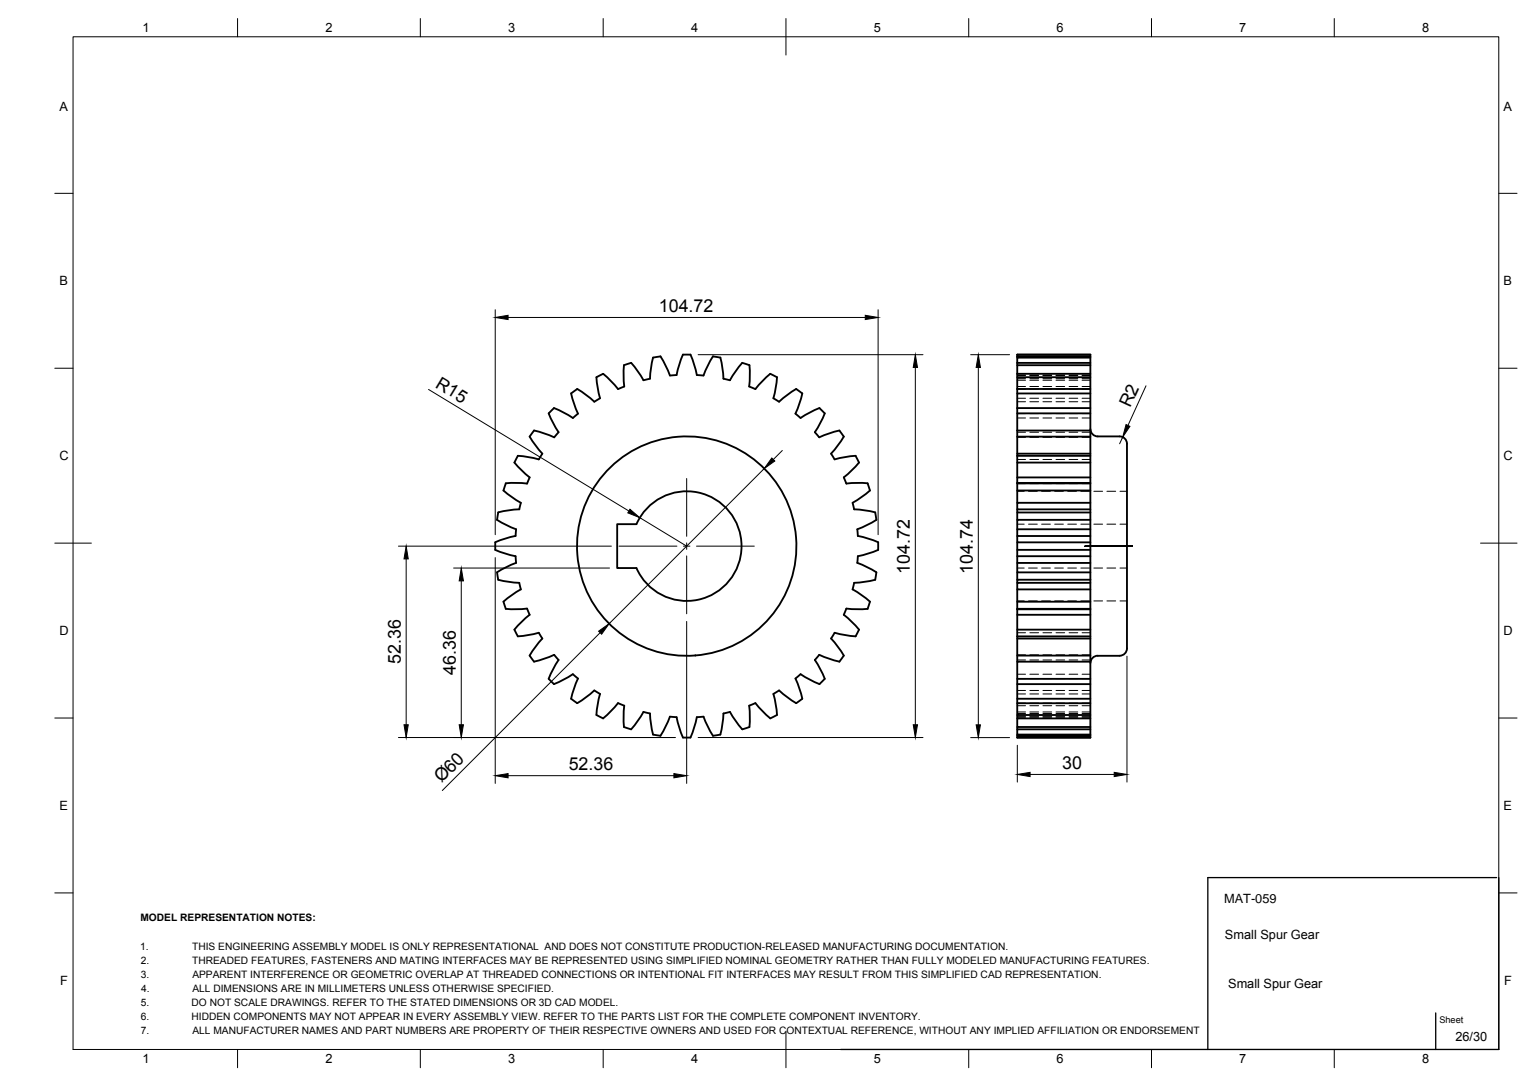
ISO-10303-21;
HEADER;
/* Generated by software containing ST-Developer
 * from STEP Tools, Inc. (www.steptools.com) 
 */

FILE_DESCRIPTION(
/* description */ ('', 'CAx-IF Rec.Pracs.---Representation and Presentation of Product Manufa
cturing Information (PMI)---4.0---2014-10-13'),
/* implementation_level */ '2;1');

FILE_NAME(
/* name */ 'Small Spur Gear.step',
/* time_stamp */ '2026-10-28T23:00:48+01:00',
/* author */ (''),
/* organization */ (''),
/* preprocessor_version */ 'ST-DEVELOPER v20.2',
/* originating_system */ 'Autodesk Translation Framework v15.17.0.0',
/* authorisation */ '');

FILE_SCHEMA (('AP242_MANAGED_MODEL_BASED_3D_ENGINEERING_MIM_LF { 1 0 10303 442 2 1 4 }'));
ENDSEC;

DATA;
#10=MECHANICAL_DESIGN_GEOMETRIC_PRESENTATION_REPRESENTATION('',(#997),#61811);
#908=TOROIDAL_SURFACE('',#36745,28.,2.);
#909=TOROIDAL_SURFACE('',#36754,32.,2.);
#933=SHAPE_REPRESENTATION_RELATIONSHIP('SRR','None',#61994,#958);
#958=ADVANCED_BREP_SHAPE_REPRESENTATION('',(#1036),#61807);
#997=STYLED_ITEM('',(#62149),#1036);
#1036=MANIFOLD_SOLID_BREP('Body1',#33827);
#1589=CYLINDRICAL_SURFACE('',#36750,30.);
#1590=CYLINDRICAL_SURFACE('',#36920,15.);
#1591=CYLINDRICAL_SURFACE('',#36923,46.875);
#1592=CYLINDRICAL_SURFACE('',#36925,27.0484525317045);
#1593=CYLINDRICAL_SURFACE('',#36927,27.0484525317045);
#1594=CYLINDRICAL_SURFACE('',#36929,46.875);
#1595=CYLINDRICAL_SURFACE('',#36931,27.0484525317045);
#1596=CYLINDRICAL_SURFACE('',#36933,27.0484525317045);
#1597=CYLINDRICAL_SURFACE('',#36935,46.875);
#1598=CYLINDRICAL_SURFACE('',#36937,27.0484525317045);
#1599=CYLINDRICAL_SURFACE('',#36939,27.0484525317045);
#1600=CYLINDRICAL_SURFACE('',#36941,46.875);
#1601=CYLINDRICAL_SURFACE('',#36943,27.0484525317045);
#1602=CYLINDRICAL_SURFACE('',#36945,27.0484525317045);
#1603=CYLINDRICAL_SURFACE('',#36947,46.875);
#1604=CYLINDRICAL_SURFACE('',#36949,27.0484525317045);
#1605=CYLINDRICAL_SURFACE('',#36951,27.0484525317045);
#1606=CYLINDRICAL_SURFACE('',#36953,46.875);
#1607=CYLINDRICAL_SURFACE('',#36955,27.0484525317045);
#1608=CYLINDRICAL_SURFACE('',#36957,27.0484525317045);
#1609=CYLINDRICAL_SURFACE('',#36959,46.875);
#1610=CYLINDRICAL_SURFACE('',#36961,27.0484525317045);
#1611=CYLINDRICAL_SURFACE('',#36963,27.0484525317045);
#1612=CYLINDRICAL_SURFACE('',#36965,46.875);
#1613=CYLINDRICAL_SURFACE('',#36967,27.0484525317045);
#1614=CYLINDRICAL_SURFACE('',#36969,27.0484525317045);
#1615=CYLINDRICAL_SURFACE('',#36971,46.875);
#1616=CYLINDRICAL_SURFACE('',#36973,27.0484525317045);
#1617=CYLINDRICAL_SURFACE('',#36975,27.0484525317045);
#1618=CYLINDRICAL_SURFACE('',#36977,46.875);
#1619=CYLINDRICAL_SURFACE('',#36979,27.0484525317045);
#1620=CYLINDRICAL_SURFACE('',#36981,27.0484525317045);
#1621=CYLINDRICAL_SURFACE('',#36983,46.875);
#1622=CYLINDRICAL_SURFACE('',#36985,27.0484525317045);
#1623=CYLINDRICAL_SURFACE('',#36987,27.0484525317045);
#1624=CYLINDRICAL_SURFACE('',#36989,46.875);
#1625=CYLINDRICAL_SURFACE('',#36991,27.0484525317045);
#1626=CYLINDRICAL_SURFACE('',#36993,27.0484525317045);
#1627=CYLINDRICAL_SURFACE('',#36995,46.875);
#1628=CYLINDRICAL_SURFACE('',#36997,27.0484525317045);
#1629=CYLINDRICAL_SURFACE('',#36999,27.0484525317045);
#1630=CYLINDRICAL_SURFACE('',#37001,46.875);
#1631=CYLINDRICAL_SURFACE('',#37003,27.0484525317045);
#1632=CYLINDRICAL_SURFACE('',#37005,27.0484525317045);
#1633=CYLINDRICAL_SURFACE('',#37007,46.875);
#1634=CYLINDRICAL_SURFACE('',#37009,27.0484525317045);
#1635=CYLINDRICAL_SURFACE('',#37011,27.0484525317045);
#1636=CYLINDRICAL_SURFACE('',#37013,46.875);
#1637=CYLINDRICAL_SURFACE('',#37015,27.0484525317045);
#1638=CYLINDRICAL_SURFACE('',#37017,27.0484525317045);
#1639=CYLINDRICAL_SURFACE('',#37019,46.875);
#1640=CYLINDRICAL_SURFACE('',#37021,27.0484525317045);
#1641=CYLINDRICAL_SURFACE('',#37023,27.0484525317045);
#1642=CYLINDRICAL_SURFACE('',#37025,46.875);
#1643=CYLINDRICAL_SURFACE('',#37027,27.0484525317045);
#1644=CYLINDRICAL_SURFACE('',#37029,27.0484525317045);
#1645=CYLINDRICAL_SURFACE('',#37031,46.875);
#1646=CYLINDRICAL_SURFACE('',#37033,27.0484525317045);
#1647=CYLINDRICAL_SURFACE('',#37035,27.0484525317045);
#1648=CYLINDRICAL_SURFACE('',#37037,46.875);
#1649=CYLINDRICAL_SURFACE('',#37039,27.0484525317045);
#1650=CYLINDRICAL_SURFACE('',#37041,27.0484525317045);
#1651=CYLINDRICAL_SURFACE('',#37043,46.875);
#1652=CYLINDRICAL_SURFACE('',#37045,27.0484525317045);
#1653=CYLINDRICAL_SURFACE('',#37047,27.0484525317045);
#1654=CYLINDRICAL_SURFACE('',#37049,46.875);
#1655=CYLINDRICAL_SURFACE('',#37051,27.0484525317045);
#1656=CYLINDRICAL_SURFACE('',#37053,27.0484525317045);
#1657=CYLINDRICAL_SURFACE('',#37055,46.875);
#1658=CYLINDRICAL_SURFACE('',#37057,27.0484525317045);
#1659=CYLINDRICAL_SURFACE('',#37059,27.0484525317045);
#1660=CYLINDRICAL_SURFACE('',#37061,46.875);
#1661=CYLINDRICAL_SURFACE('',#37063,27.0484525317045);
#1662=CYLINDRICAL_SURFACE('',#37065,27.0484525317045);
#1663=CYLINDRICAL_SURFACE('',#37067,46.875);
#1664=CYLINDRICAL_SURFACE('',#37069,27.0484525317045);
#1665=CYLINDRICAL_SURFACE('',#37071,27.0484525317045);
#1666=CYLINDRICAL_SURFACE('',#37073,46.875);
#1667=CYLINDRICAL_SURFACE('',#37075,27.0484525317045);
#1668=CYLINDRICAL_SURFACE('',#37077,27.0484525317045);
#1669=CYLINDRICAL_SURFACE('',#37079,46.875);
#1670=CYLINDRICAL_SURFACE('',#37081,27.0484525317045);
#1671=CYLINDRICAL_SURFACE('',#37083,27.0484525317045);
#1672=CYLINDRICAL_SURFACE('',#37085,46.875);
#1673=CYLINDRICAL_SURFACE('',#37087,27.0484525317045);
#1674=CYLINDRICAL_SURFACE('',#37089,27.0484525317045);
#1675=CYLINDRICAL_SURFACE('',#37091,46.875);
#1676=CYLINDRICAL_SURFACE('',#37093,27.0484525317045);
#1677=CYLINDRICAL_SURFACE('',#37095,27.0484525317045);
#1678=CYLINDRICAL_SURFACE('',#37097,46.875);
#1679=CYLINDRICAL_SURFACE('',#37099,27.0484525317045);
#1680=CYLINDRICAL_SURFACE('',#37101,27.0484525317045);
#1681=CYLINDRICAL_SURFACE('',#37103,46.875);
#1682=CYLINDRICAL_SURFACE('',#37105,27.0484525317045);
#1683=CYLINDRICAL_SURFACE('',#37107,27.0484525317045);
#1684=CYLINDRICAL_SURFACE('',#37109,46.875);
#1685=CYLINDRICAL_SURFACE('',#37111,27.0484525317045);
#1686=CYLINDRICAL_SURFACE('',#37113,27.0484525317045);
#1687=CYLINDRICAL_SURFACE('',#37115,46.875);
#1688=CYLINDRICAL_SURFACE('',#37117,27.0484525317045);
#1689=CYLINDRICAL_SURFACE('',#37119,27.0484525317045);
#1690=CYLINDRICAL_SURFACE('',#37121,46.875);
#1691=CYLINDRICAL_SURFACE('',#37123,27.0484525317045);
#1692=CYLINDRICAL_SURFACE('',#37125,27.0484525317045);
#1693=CYLINDRICAL_SURFACE('',#37127,46.875);
#1694=CYLINDRICAL_SURFACE('',#37129,27.0484525317045);
#1695=CYLINDRICAL_SURFACE('',#37131,27.0484525317045);
#1696=CYLINDRICAL_SURFACE('',#37133,46.875);
#1697=CYLINDRICAL_SURFACE('',#37135,27.0484525317045);
#1698=CYLINDRICAL_SURFACE('',#37137,27.0484525317045);
#1699=CYLINDRICAL_SURFACE('',#37139,46.875);
#1700=CYLINDRICAL_SURFACE('',#37141,27.0484525317045);
#1701=CYLINDRICAL_SURFACE('',#37143,27.0484525317045);
#1702=CYLINDRICAL_SURFACE('',#37145,46.875);
#1703=CYLINDRICAL_SURFACE('',#37147,27.0484525317045);
#1704=CYLINDRICAL_SURFACE('',#37149,27.0484525317045);
#1705=CYLINDRICAL_SURFACE('',#37151,46.875);
#1706=CYLINDRICAL_SURFACE('',#37153,27.0484525317045);
#1707=CYLINDRICAL_SURFACE('',#37155,27.0484525317045);
#1708=CYLINDRICAL_SURFACE('',#37157,52.37069718);
#1709=CYLINDRICAL_SURFACE('',#37159,52.37069718);
#1710=CYLINDRICAL_SURFACE('',#37161,52.37069718);
#1711=CYLINDRICAL_SURFACE('',#37163,52.37069718);
#1712=CYLINDRICAL_SURFACE('',#37165,52.37069718);
#1713=CYLINDRICAL_SURFACE('',#37167,52.37069718);
#1714=CYLINDRICAL_SURFACE('',#37169,52.37069718);
#1715=CYLINDRICAL_SURFACE('',#37171,52.37069718);
#1716=CYLINDRICAL_SURFACE('',#37173,52.37069718);
#1717=CYLINDRICAL_SURFACE('',#37175,52.37069718);
#1718=CYLINDRICAL_SURFACE('',#37177,52.37069718);
#1719=CYLINDRICAL_SURFACE('',#37179,52.37069718);
#1720=CYLINDRICAL_SURFACE('',#37181,52.37069718);
#1721=CYLINDRICAL_SURFACE('',#37183,52.37069718);
#1722=CYLINDRICAL_SURFACE('',#37185,52.37069718);
#1723=CYLINDRICAL_SURFACE('',#37187,52.37069718);
#1724=CYLINDRICAL_SURFACE('',#37189,52.37069718);
#1725=CYLINDRICAL_SURFACE('',#37191,52.37069718);
#1726=CYLINDRICAL_SURFACE('',#37193,52.37069718);
#1727=CYLINDRICAL_SURFACE('',#37195,52.37069718);
#1728=CYLINDRICAL_SURFACE('',#37197,52.37069718);
#1729=CYLINDRICAL_SURFACE('',#37199,52.37069718);
#1730=CYLINDRICAL_SURFACE('',#37201,52.37069718);
#1731=CYLINDRICAL_SURFACE('',#37203,52.37069718);
#1732=CYLINDRICAL_SURFACE('',#37205,52.37069718);
#1733=CYLINDRICAL_SURFACE('',#37207,52.37069718);
#1734=CYLINDRICAL_SURFACE('',#37209,52.37069718);
#1735=CYLINDRICAL_SURFACE('',#37211,52.37069718);
#1736=CYLINDRICAL_SURFACE('',#37213,52.37069718);
#1737=CYLINDRICAL_SURFACE('',#37215,52.37069718);
#1738=CYLINDRICAL_SURFACE('',#37217,52.37069718);
#1739=CYLINDRICAL_SURFACE('',#37219,52.37069718);
#1740=CYLINDRICAL_SURFACE('',#37221,52.37069718);
#1741=CYLINDRICAL_SURFACE('',#37223,52.37069718);
#1742=CYLINDRICAL_SURFACE('',#37225,52.37069718);
#1743=CYLINDRICAL_SURFACE('',#37227,52.37069718);
#1744=CYLINDRICAL_SURFACE('',#37229,52.37069718);
#1745=CYLINDRICAL_SURFACE('',#37231,52.37069718);
#1746=CYLINDRICAL_SURFACE('',#37233,52.37069718);
#1747=CYLINDRICAL_SURFACE('',#37235,46.875);
#1748=CYLINDRICAL_SURFACE('',#37237,27.0484525317045);
#1749=CYLINDRICAL_SURFACE('',#37239,27.0484525317045);
#1750=CYLINDRICAL_SURFACE('',#37241,52.37069718);
#2134=FACE_BOUND('',#7611,.T.);
#2135=FACE_BOUND('',#7614,.T.);
#2136=FACE_BOUND('',#7780,.T.);
#3518=CIRCLE('',#36746,28.);
#3519=CIRCLE('',#36747,2.);
#3520=CIRCLE('',#36748,30.);
#3521=CIRCLE('',#36749,30.);
#3522=CIRCLE('',#36751,30.);
#3523=CIRCLE('',#36753,15.);
#3524=CIRCLE('',#36755,32.);
#3525=CIRCLE('',#36756,2.);
#3526=CIRCLE('',#36758,27.0484525317045);
#3527=CIRCLE('',#36759,46.875);
#3528=CIRCLE('',#36760,27.0484525317045);
#3529=CIRCLE('',#36761,52.37069718);
#3530=CIRCLE('',#36762,27.0484525317045);
#3531=CIRCLE('',#36763,46.875);
#3532=CIRCLE('',#36764,27.0484525317045);
#3533=CIRCLE('',#36765,52.37069718);
#3534=CIRCLE('',#36766,27.0484525317045);
#3535=CIRCLE('',#36767,46.875);
#3536=CIRCLE('',#36768,27.0484525317045);
#3537=CIRCLE('',#36769,52.37069718);
#3538=CIRCLE('',#36770,27.0484525317045);
#3539=CIRCLE('',#36771,46.875);
#3540=CIRCLE('',#36772,27.0484525317045);
#3541=CIRCLE('',#36773,52.37069718);
#3542=CIRCLE('',#36774,27.0484525317045);
#3543=CIRCLE('',#36775,46.875);
#3544=CIRCLE('',#36776,27.0484525317045);
#3545=CIRCLE('',#36777,52.37069718);
#3546=CIRCLE('',#36778,27.0484525317045);
#3547=CIRCLE('',#36779,46.875);
#3548=CIRCLE('',#36780,27.0484525317045);
#3549=CIRCLE('',#36781,52.37069718);
#3550=CIRCLE('',#36782,27.0484525317045);
#3551=CIRCLE('',#36783,46.875);
#3552=CIRCLE('',#36784,27.0484525317045);
#3553=CIRCLE('',#36785,52.37069718);
#3554=CIRCLE('',#36786,27.0484525317045);
#3555=CIRCLE('',#36787,46.875);
#3556=CIRCLE('',#36788,27.0484525317045);
#3557=CIRCLE('',#36789,52.37069718);
#3558=CIRCLE('',#36790,27.0484525317045);
#3559=CIRCLE('',#36791,46.875);
#3560=CIRCLE('',#36792,27.0484525317045);
#3561=CIRCLE('',#36793,52.37069718);
#3562=CIRCLE('',#36794,27.0484525317045);
#3563=CIRCLE('',#36795,46.875);
#3564=CIRCLE('',#36796,27.0484525317045);
#3565=CIRCLE('',#36797,52.37069718);
#3566=CIRCLE('',#36798,27.0484525317045);
#3567=CIRCLE('',#36799,46.875);
#3568=CIRCLE('',#36800,27.0484525317045);
#3569=CIRCLE('',#36801,52.37069718);
#3570=CIRCLE('',#36802,27.0484525317045);
#3571=CIRCLE('',#36803,46.875);
#3572=CIRCLE('',#36804,27.0484525317045);
#3573=CIRCLE('',#36805,52.37069718);
#3574=CIRCLE('',#36806,27.0484525317045);
#3575=CIRCLE('',#36807,46.875);
#3576=CIRCLE('',#36808,27.0484525317045);
#3577=CIRCLE('',#36809,52.37069718);
#3578=CIRCLE('',#36810,27.0484525317045);
#3579=CIRCLE('',#36811,46.875);
#3580=CIRCLE('',#36812,27.0484525317045);
#3581=CIRCLE('',#36813,52.37069718);
#3582=CIRCLE('',#36814,27.0484525317045);
#3583=CIRCLE('',#36815,46.875);
#3584=CIRCLE('',#36816,27.0484525317045);
#3585=CIRCLE('',#36817,52.37069718);
#3586=CIRCLE('',#36818,27.0484525317045);
#3587=CIRCLE('',#36819,46.875);
#3588=CIRCLE('',#36820,27.0484525317045);
#3589=CIRCLE('',#36821,52.37069718);
#3590=CIRCLE('',#36822,27.0484525317045);
#3591=CIRCLE('',#36823,46.875);
#3592=CIRCLE('',#36824,27.0484525317045);
#3593=CIRCLE('',#36825,52.37069718);
#3594=CIRCLE('',#36826,27.0484525317045);
#3595=CIRCLE('',#36827,46.875);
#3596=CIRCLE('',#36828,27.0484525317045);
#3597=CIRCLE('',#36829,52.37069718);
#3598=CIRCLE('',#36830,27.0484525317045);
#3599=CIRCLE('',#36831,46.875);
#3600=CIRCLE('',#36832,27.0484525317045);
#3601=CIRCLE('',#36833,52.37069718);
#3602=CIRCLE('',#36834,27.0484525317045);
#3603=CIRCLE('',#36835,46.875);
#3604=CIRCLE('',#36836,27.0484525317045);
#3605=CIRCLE('',#36837,52.37069718);
#3606=CIRCLE('',#36838,27.0484525317045);
#3607=CIRCLE('',#36839,46.875);
#3608=CIRCLE('',#36840,27.0484525317045);
#3609=CIRCLE('',#36841,52.37069718);
#3610=CIRCLE('',#36842,27.0484525317045);
#3611=CIRCLE('',#36843,46.875);
#3612=CIRCLE('',#36844,27.0484525317045);
#3613=CIRCLE('',#36845,52.37069718);
#3614=CIRCLE('',#36846,27.0484525317045);
#3615=CIRCLE('',#36847,46.875);
#3616=CIRCLE('',#36848,27.0484525317045);
#3617=CIRCLE('',#36849,52.37069718);
#3618=CIRCLE('',#36850,27.0484525317045);
#3619=CIRCLE('',#36851,46.875);
#3620=CIRCLE('',#36852,27.0484525317045);
#3621=CIRCLE('',#36853,52.37069718);
#3622=CIRCLE('',#36854,27.0484525317045);
#3623=CIRCLE('',#36855,46.875);
#3624=CIRCLE('',#36856,27.0484525317045);
#3625=CIRCLE('',#36857,52.37069718);
#3626=CIRCLE('',#36858,27.0484525317045);
#3627=CIRCLE('',#36859,46.875);
#3628=CIRCLE('',#36860,27.0484525317045);
#3629=CIRCLE('',#36861,52.37069718);
#3630=CIRCLE('',#36862,27.0484525317045);
#3631=CIRCLE('',#36863,46.875);
#3632=CIRCLE('',#36864,27.0484525317045);
#3633=CIRCLE('',#36865,52.37069718);
#3634=CIRCLE('',#36866,27.0484525317045);
#3635=CIRCLE('',#36867,46.875);
#3636=CIRCLE('',#36868,27.0484525317045);
#3637=CIRCLE('',#36869,52.37069718);
#3638=CIRCLE('',#36870,27.0484525317045);
#3639=CIRCLE('',#36871,46.875);
#3640=CIRCLE('',#36872,27.0484525317045);
#3641=CIRCLE('',#36873,52.37069718);
#3642=CIRCLE('',#36874,27.0484525317045);
#3643=CIRCLE('',#36875,46.875);
#3644=CIRCLE('',#36876,27.0484525317045);
#3645=CIRCLE('',#36877,52.37069718);
#3646=CIRCLE('',#36878,27.0484525317045);
#3647=CIRCLE('',#36879,46.875);
#3648=CIRCLE('',#36880,27.0484525317045);
#3649=CIRCLE('',#36881,52.37069718);
#3650=CIRCLE('',#36882,27.0484525317045);
#3651=CIRCLE('',#36883,46.875);
#3652=CIRCLE('',#36884,27.0484525317045);
#3653=CIRCLE('',#36885,52.37069718);
#3654=CIRCLE('',#36886,27.0484525317045);
#3655=CIRCLE('',#36887,46.875);
#3656=CIRCLE('',#36888,27.0484525317045);
#3657=CIRCLE('',#36889,52.37069718);
#3658=CIRCLE('',#36890,27.0484525317045);
#3659=CIRCLE('',#36891,46.875);
#3660=CIRCLE('',#36892,27.0484525317045);
#3661=CIRCLE('',#36893,52.37069718);
#3662=CIRCLE('',#36894,27.0484525317045);
#3663=CIRCLE('',#36895,46.875);
#3664=CIRCLE('',#36896,27.0484525317045);
#3665=CIRCLE('',#36897,52.37069718);
#3666=CIRCLE('',#36898,27.0484525317045);
#3667=CIRCLE('',#36899,46.875);
#3668=CIRCLE('',#36900,27.0484525317045);
#3669=CIRCLE('',#36901,52.37069718);
#3670=CIRCLE('',#36902,27.0484525317045);
#3671=CIRCLE('',#36903,46.875);
#3672=CIRCLE('',#36904,27.0484525317045);
#3673=CIRCLE('',#36905,52.37069718);
#3674=CIRCLE('',#36906,27.0484525317045);
#3675=CIRCLE('',#36907,46.875);
#3676=CIRCLE('',#36908,27.0484525317045);
#3677=CIRCLE('',#36909,52.37069718);
#3678=CIRCLE('',#36910,27.0484525317045);
#3679=CIRCLE('',#36911,46.875);
#3680=CIRCLE('',#36912,27.0484525317045);
#3681=CIRCLE('',#36913,52.37069718);
#3682=CIRCLE('',#36914,27.0484525317045);
#3683=CIRCLE('',#36915,46.875);
#3684=CIRCLE('',#36916,27.0484525317045);
#3685=CIRCLE('',#36917,52.37069718);
#3686=CIRCLE('',#36921,15.);
#3687=CIRCLE('',#36924,46.875);
#3688=CIRCLE('',#36926,27.0484525317045);
#3689=CIRCLE('',#36928,27.0484525317045);
#3690=CIRCLE('',#36930,46.875);
#3691=CIRCLE('',#36932,27.0484525317045);
#3692=CIRCLE('',#36934,27.0484525317045);
#3693=CIRCLE('',#36936,46.875);
#3694=CIRCLE('',#36938,27.0484525317045);
#3695=CIRCLE('',#36940,27.0484525317045);
#3696=CIRCLE('',#36942,46.875);
#3697=CIRCLE('',#36944,27.0484525317045);
#3698=CIRCLE('',#36946,27.0484525317045);
#3699=CIRCLE('',#36948,46.875);
#3700=CIRCLE('',#36950,27.0484525317045);
#3701=CIRCLE('',#36952,27.0484525317045);
#3702=CIRCLE('',#36954,46.875);
#3703=CIRCLE('',#36956,27.0484525317045);
#3704=CIRCLE('',#36958,27.0484525317045);
#3705=CIRCLE('',#36960,46.875);
#3706=CIRCLE('',#36962,27.0484525317045);
#3707=CIRCLE('',#36964,27.0484525317045);
#3708=CIRCLE('',#36966,46.875);
#3709=CIRCLE('',#36968,27.0484525317045);
#3710=CIRCLE('',#36970,27.0484525317045);
#3711=CIRCLE('',#36972,46.875);
#3712=CIRCLE('',#36974,27.0484525317045);
#3713=CIRCLE('',#36976,27.0484525317045);
#3714=CIRCLE('',#36978,46.875);
#3715=CIRCLE('',#36980,27.0484525317045);
#3716=CIRCLE('',#36982,27.0484525317045);
#3717=CIRCLE('',#36984,46.875);
#3718=CIRCLE('',#36986,27.0484525317045);
#3719=CIRCLE('',#36988,27.0484525317045);
#3720=CIRCLE('',#36990,46.875);
#3721=CIRCLE('',#36992,27.0484525317045);
#3722=CIRCLE('',#36994,27.0484525317045);
#3723=CIRCLE('',#36996,46.875);
#3724=CIRCLE('',#36998,27.0484525317045);
#3725=CIRCLE('',#37000,27.0484525317045);
#3726=CIRCLE('',#37002,46.875);
#3727=CIRCLE('',#37004,27.0484525317045);
#3728=CIRCLE('',#37006,27.0484525317045);
#3729=CIRCLE('',#37008,46.875);
#3730=CIRCLE('',#37010,27.0484525317045);
#3731=CIRCLE('',#37012,27.0484525317045);
#3732=CIRCLE('',#37014,46.875);
#3733=CIRCLE('',#37016,27.0484525317045);
#3734=CIRCLE('',#37018,27.0484525317045);
#3735=CIRCLE('',#37020,46.875);
#3736=CIRCLE('',#37022,27.0484525317045);
#3737=CIRCLE('',#37024,27.0484525317045);
#3738=CIRCLE('',#37026,46.875);
#3739=CIRCLE('',#37028,27.0484525317045);
#3740=CIRCLE('',#37030,27.0484525317045);
#3741=CIRCLE('',#37032,46.875);
#3742=CIRCLE('',#37034,27.0484525317045);
#3743=CIRCLE('',#37036,27.0484525317045);
#3744=CIRCLE('',#37038,46.875);
#3745=CIRCLE('',#37040,27.0484525317045);
#3746=CIRCLE('',#37042,27.0484525317045);
#3747=CIRCLE('',#37044,46.875);
#3748=CIRCLE('',#37046,27.0484525317045);
#3749=CIRCLE('',#37048,27.0484525317045);
#3750=CIRCLE('',#37050,46.875);
#3751=CIRCLE('',#37052,27.0484525317045);
#3752=CIRCLE('',#37054,27.0484525317045);
#3753=CIRCLE('',#37056,46.875);
#3754=CIRCLE('',#37058,27.0484525317045);
#3755=CIRCLE('',#37060,27.0484525317045);
#3756=CIRCLE('',#37062,46.875);
#3757=CIRCLE('',#37064,27.0484525317045);
#3758=CIRCLE('',#37066,27.0484525317045);
#3759=CIRCLE('',#37068,46.875);
#3760=CIRCLE('',#37070,27.0484525317045);
#3761=CIRCLE('',#37072,27.0484525317045);
#3762=CIRCLE('',#37074,46.875);
#3763=CIRCLE('',#37076,27.0484525317045);
#3764=CIRCLE('',#37078,27.0484525317045);
#3765=CIRCLE('',#37080,46.875);
#3766=CIRCLE('',#37082,27.0484525317045);
#3767=CIRCLE('',#37084,27.0484525317045);
#3768=CIRCLE('',#37086,46.875);
#3769=CIRCLE('',#37088,27.0484525317045);
#3770=CIRCLE('',#37090,27.0484525317045);
#3771=CIRCLE('',#37092,46.875);
#3772=CIRCLE('',#37094,27.0484525317045);
#3773=CIRCLE('',#37096,27.0484525317045);
#3774=CIRCLE('',#37098,46.875);
#3775=CIRCLE('',#37100,27.0484525317045);
#3776=CIRCLE('',#37102,27.0484525317045);
#3777=CIRCLE('',#37104,46.875);
#3778=CIRCLE('',#37106,27.0484525317045);
#3779=CIRCLE('',#37108,27.0484525317045);
#3780=CIRCLE('',#37110,46.875);
#3781=CIRCLE('',#37112,27.0484525317045);
#3782=CIRCLE('',#37114,27.0484525317045);
#3783=CIRCLE('',#37116,46.875);
#3784=CIRCLE('',#37118,27.0484525317045);
#3785=CIRCLE('',#37120,27.0484525317045);
#3786=CIRCLE('',#37122,46.875);
#3787=CIRCLE('',#37124,27.0484525317045);
#3788=CIRCLE('',#37126,27.0484525317045);
#3789=CIRCLE('',#37128,46.875);
#3790=CIRCLE('',#37130,27.0484525317045);
#3791=CIRCLE('',#37132,27.0484525317045);
#3792=CIRCLE('',#37134,46.875);
#3793=CIRCLE('',#37136,27.0484525317045);
#3794=CIRCLE('',#37138,27.0484525317045);
#3795=CIRCLE('',#37140,46.875);
#3796=CIRCLE('',#37142,27.0484525317045);
#3797=CIRCLE('',#37144,27.0484525317045);
#3798=CIRCLE('',#37146,46.875);
#3799=CIRCLE('',#37148,27.0484525317045);
#3800=CIRCLE('',#37150,27.0484525317045);
#3801=CIRCLE('',#37152,46.875);
#3802=CIRCLE('',#37154,27.0484525317045);
#3803=CIRCLE('',#37156,27.0484525317045);
#3804=CIRCLE('',#37158,52.37069718);
#3805=CIRCLE('',#37160,52.37069718);
#3806=CIRCLE('',#37162,52.37069718);
#3807=CIRCLE('',#37164,52.37069718);
#3808=CIRCLE('',#37166,52.37069718);
#3809=CIRCLE('',#37168,52.37069718);
#3810=CIRCLE('',#37170,52.37069718);
#3811=CIRCLE('',#37172,52.37069718);
#3812=CIRCLE('',#37174,52.37069718);
#3813=CIRCLE('',#37176,52.37069718);
#3814=CIRCLE('',#37178,52.37069718);
#3815=CIRCLE('',#37180,52.37069718);
#3816=CIRCLE('',#37182,52.37069718);
#3817=CIRCLE('',#37184,52.37069718);
#3818=CIRCLE('',#37186,52.37069718);
#3819=CIRCLE('',#37188,52.37069718);
#3820=CIRCLE('',#37190,52.37069718);
#3821=CIRCLE('',#37192,52.37069718);
#3822=CIRCLE('',#37194,52.37069718);
#3823=CIRCLE('',#37196,52.37069718);
#3824=CIRCLE('',#37198,52.37069718);
#3825=CIRCLE('',#37200,52.37069718);
#3826=CIRCLE('',#37202,52.37069718);
#3827=CIRCLE('',#37204,52.37069718);
#3828=CIRCLE('',#37206,52.37069718);
#3829=CIRCLE('',#37208,52.37069718);
#3830=CIRCLE('',#37210,52.37069718);
#3831=CIRCLE('',#37212,52.37069718);
#3832=CIRCLE('',#37214,52.37069718);
#3833=CIRCLE('',#37216,52.37069718);
#3834=CIRCLE('',#37218,52.37069718);
#3835=CIRCLE('',#37220,52.37069718);
#3836=CIRCLE('',#37222,52.37069718);
#3837=CIRCLE('',#37224,52.37069718);
#3838=CIRCLE('',#37226,52.37069718);
#3839=CIRCLE('',#37228,52.37069718);
#3840=CIRCLE('',#37230,52.37069718);
#3841=CIRCLE('',#37232,52.37069718);
#3842=CIRCLE('',#37234,52.37069718);
#3843=CIRCLE('',#37236,46.875);
#3844=CIRCLE('',#37238,27.0484525317045);
#3845=CIRCLE('',#37240,27.0484525317045);
#3846=CIRCLE('',#37242,52.37069718);
#5474=FACE_OUTER_BOUND('',#7608,.T.);
#5475=FACE_OUTER_BOUND('',#7609,.T.);
#5476=FACE_OUTER_BOUND('',#7610,.T.);
#5477=FACE_OUTER_BOUND('',#7612,.T.);
#5478=FACE_OUTER_BOUND('',#7613,.T.);
#5479=FACE_OUTER_BOUND('',#7615,.T.);
#5480=FACE_OUTER_BOUND('',#7616,.T.);
#5481=FACE_OUTER_BOUND('',#7617,.T.);
#5482=FACE_OUTER_BOUND('',#7618,.T.);
#5483=FACE_OUTER_BOUND('',#7619,.T.);
#5484=FACE_OUTER_BOUND('',#7620,.T.);
#5485=FACE_OUTER_BOUND('',#7621,.T.);
#5486=FACE_OUTER_BOUND('',#7622,.T.);
#5487=FACE_OUTER_BOUND('',#7623,.T.);
#5488=FACE_OUTER_BOUND('',#7624,.T.);
#5489=FACE_OUTER_BOUND('',#7625,.T.);
#5490=FACE_OUTER_BOUND('',#7626,.T.);
#5491=FACE_OUTER_BOUND('',#7627,.T.);
#5492=FACE_OUTER_BOUND('',#7628,.T.);
#5493=FACE_OUTER_BOUND('',#7629,.T.);
#5494=FACE_OUTER_BOUND('',#7630,.T.);
#5495=FACE_OUTER_BOUND('',#7631,.T.);
#5496=FACE_OUTER_BOUND('',#7632,.T.);
#5497=FACE_OUTER_BOUND('',#7633,.T.);
#5498=FACE_OUTER_BOUND('',#7634,.T.);
#5499=FACE_OUTER_BOUND('',#7635,.T.);
#5500=FACE_OUTER_BOUND('',#7636,.T.);
#5501=FACE_OUTER_BOUND('',#7637,.T.);
#5502=FACE_OUTER_BOUND('',#7638,.T.);
#5503=FACE_OUTER_BOUND('',#7639,.T.);
#5504=FACE_OUTER_BOUND('',#7640,.T.);
#5505=FACE_OUTER_BOUND('',#7641,.T.);
#5506=FACE_OUTER_BOUND('',#7642,.T.);
#5507=FACE_OUTER_BOUND('',#7643,.T.);
#5508=FACE_OUTER_BOUND('',#7644,.T.);
#5509=FACE_OUTER_BOUND('',#7645,.T.);
#5510=FACE_OUTER_BOUND('',#7646,.T.);
#5511=FACE_OUTER_BOUND('',#7647,.T.);
#5512=FACE_OUTER_BOUND('',#7648,.T.);
#5513=FACE_OUTER_BOUND('',#7649,.T.);
#5514=FACE_OUTER_BOUND('',#7650,.T.);
#5515=FACE_OUTER_BOUND('',#7651,.T.);
#5516=FACE_OUTER_BOUND('',#7652,.T.);
#5517=FACE_OUTER_BOUND('',#7653,.T.);
#5518=FACE_OUTER_BOUND('',#7654,.T.);
#5519=FACE_OUTER_BOUND('',#7655,.T.);
#5520=FACE_OUTER_BOUND('',#7656,.T.);
#5521=FACE_OUTER_BOUND('',#7657,.T.);
#5522=FACE_OUTER_BOUND('',#7658,.T.);
#5523=FACE_OUTER_BOUND('',#7659,.T.);
#5524=FACE_OUTER_BOUND('',#7660,.T.);
#5525=FACE_OUTER_BOUND('',#7661,.T.);
#5526=FACE_OUTER_BOUND('',#7662,.T.);
#5527=FACE_OUTER_BOUND('',#7663,.T.);
#5528=FACE_OUTER_BOUND('',#7664,.T.);
#5529=FACE_OUTER_BOUND('',#7665,.T.);
#5530=FACE_OUTER_BOUND('',#7666,.T.);
#5531=FACE_OUTER_BOUND('',#7667,.T.);
#5532=FACE_OUTER_BOUND('',#7668,.T.);
#5533=FACE_OUTER_BOUND('',#7669,.T.);
#5534=FACE_OUTER_BOUND('',#7670,.T.);
#5535=FACE_OUTER_BOUND('',#7671,.T.);
#5536=FACE_OUTER_BOUND('',#7672,.T.);
#5537=FACE_OUTER_BOUND('',#7673,.T.);
#5538=FACE_OUTER_BOUND('',#7674,.T.);
#5539=FACE_OUTER_BOUND('',#7675,.T.);
#5540=FACE_OUTER_BOUND('',#7676,.T.);
#5541=FACE_OUTER_BOUND('',#7677,.T.);
#5542=FACE_OUTER_BOUND('',#7678,.T.);
#5543=FACE_OUTER_BOUND('',#7679,.T.);
#5544=FACE_OUTER_BOUND('',#7680,.T.);
#5545=FACE_OUTER_BOUND('',#7681,.T.);
#5546=FACE_OUTER_BOUND('',#7682,.T.);
#5547=FACE_OUTER_BOUND('',#7683,.T.);
#5548=FACE_OUTER_BOUND('',#7684,.T.);
#5549=FACE_OUTER_BOUND('',#7685,.T.);
#5550=FACE_OUTER_BOUND('',#7686,.T.);
#5551=FACE_OUTER_BOUND('',#7687,.T.);
#5552=FACE_OUTER_BOUND('',#7688,.T.);
#5553=FACE_OUTER_BOUND('',#7689,.T.);
#5554=FACE_OUTER_BOUND('',#7690,.T.);
#5555=FACE_OUTER_BOUND('',#7691,.T.);
#5556=FACE_OUTER_BOUND('',#7692,.T.);
#5557=FACE_OUTER_BOUND('',#7693,.T.);
#5558=FACE_OUTER_BOUND('',#7694,.T.);
#5559=FACE_OUTER_BOUND('',#7695,.T.);
#5560=FACE_OUTER_BOUND('',#7696,.T.);
#5561=FACE_OUTER_BOUND('',#7697,.T.);
#5562=FACE_OUTER_BOUND('',#7698,.T.);
#5563=FACE_OUTER_BOUND('',#7699,.T.);
#5564=FACE_OUTER_BOUND('',#7700,.T.);
#5565=FACE_OUTER_BOUND('',#7701,.T.);
#5566=FACE_OUTER_BOUND('',#7702,.T.);
#5567=FACE_OUTER_BOUND('',#7703,.T.);
#5568=FACE_OUTER_BOUND('',#7704,.T.);
#5569=FACE_OUTER_BOUND('',#7705,.T.);
#5570=FACE_OUTER_BOUND('',#7706,.T.);
#5571=FACE_OUTER_BOUND('',#7707,.T.);
#5572=FACE_OUTER_BOUND('',#7708,.T.);
#5573=FACE_OUTER_BOUND('',#7709,.T.);
#5574=FACE_OUTER_BOUND('',#7710,.T.);
#5575=FACE_OUTER_BOUND('',#7711,.T.);
#5576=FACE_OUTER_BOUND('',#7712,.T.);
#5577=FACE_OUTER_BOUND('',#7713,.T.);
#5578=FACE_OUTER_BOUND('',#7714,.T.);
#5579=FACE_OUTER_BOUND('',#7715,.T.);
#5580=FACE_OUTER_BOUND('',#7716,.T.);
#5581=FACE_OUTER_BOUND('',#7717,.T.);
#5582=FACE_OUTER_BOUND('',#7718,.T.);
#5583=FACE_OUTER_BOUND('',#7719,.T.);
#5584=FACE_OUTER_BOUND('',#7720,.T.);
#5585=FACE_OUTER_BOUND('',#7721,.T.);
#5586=FACE_OUTER_BOUND('',#7722,.T.);
#5587=FACE_OUTER_BOUND('',#7723,.T.);
#5588=FACE_OUTER_BOUND('',#7724,.T.);
#5589=FACE_OUTER_BOUND('',#7725,.T.);
#5590=FACE_OUTER_BOUND('',#7726,.T.);
#5591=FACE_OUTER_BOUND('',#7727,.T.);
#5592=FACE_OUTER_BOUND('',#7728,.T.);
#5593=FACE_OUTER_BOUND('',#7729,.T.);
#5594=FACE_OUTER_BOUND('',#7730,.T.);
#5595=FACE_OUTER_BOUND('',#7731,.T.);
#5596=FACE_OUTER_BOUND('',#7732,.T.);
#5597=FACE_OUTER_BOUND('',#7733,.T.);
#5598=FACE_OUTER_BOUND('',#7734,.T.);
#5599=FACE_OUTER_BOUND('',#7735,.T.);
#5600=FACE_OUTER_BOUND('',#7736,.T.);
#5601=FACE_OUTER_BOUND('',#7737,.T.);
#5602=FACE_OUTER_BOUND('',#7738,.T.);
#5603=FACE_OUTER_BOUND('',#7739,.T.);
#5604=FACE_OUTER_BOUND('',#7740,.T.);
#5605=FACE_OUTER_BOUND('',#7741,.T.);
#5606=FACE_OUTER_BOUND('',#7742,.T.);
#5607=FACE_OUTER_BOUND('',#7743,.T.);
#5608=FACE_OUTER_BOUND('',#7744,.T.);
#5609=FACE_OUTER_BOUND('',#7745,.T.);
#5610=FACE_OUTER_BOUND('',#7746,.T.);
#5611=FACE_OUTER_BOUND('',#7747,.T.);
#5612=FACE_OUTER_BOUND('',#7748,.T.);
#5613=FACE_OUTER_BOUND('',#7749,.T.);
#5614=FACE_OUTER_BOUND('',#7750,.T.);
#5615=FACE_OUTER_BOUND('',#7751,.T.);
#5616=FACE_OUTER_BOUND('',#7752,.T.);
#5617=FACE_OUTER_BOUND('',#7753,.T.);
#5618=FACE_OUTER_BOUND('',#7754,.T.);
#5619=FACE_OUTER_BOUND('',#7755,.T.);
#5620=FACE_OUTER_BOUND('',#7756,.T.);
#5621=FACE_OUTER_BOUND('',#7757,.T.);
#5622=FACE_OUTER_BOUND('',#7758,.T.);
#5623=FACE_OUTER_BOUND('',#7759,.T.);
#5624=FACE_OUTER_BOUND('',#7760,.T.);
#5625=FACE_OUTER_BOUND('',#7761,.T.);
#5626=FACE_OUTER_BOUND('',#7762,.T.);
#5627=FACE_OUTER_BOUND('',#7763,.T.);
#5628=FACE_OUTER_BOUND('',#7764,.T.);
#5629=FACE_OUTER_BOUND('',#7765,.T.);
#5630=FACE_OUTER_BOUND('',#7766,.T.);
#5631=FACE_OUTER_BOUND('',#7767,.T.);
#5632=FACE_OUTER_BOUND('',#7768,.T.);
#5633=FACE_OUTER_BOUND('',#7769,.T.);
#5634=FACE_OUTER_BOUND('',#7770,.T.);
#5635=FACE_OUTER_BOUND('',#7771,.T.);
#5636=FACE_OUTER_BOUND('',#7772,.T.);
#5637=FACE_OUTER_BOUND('',#7773,.T.);
#5638=FACE_OUTER_BOUND('',#7774,.T.);
#5639=FACE_OUTER_BOUND('',#7775,.T.);
#5640=FACE_OUTER_BOUND('',#7776,.T.);
#5641=FACE_OUTER_BOUND('',#7777,.T.);
#5642=FACE_OUTER_BOUND('',#7778,.T.);
#5643=FACE_OUTER_BOUND('',#7779,.T.);
#7608=EDGE_LOOP('',(#27770,#27771,#27772,#27773,#27774));
#7609=EDGE_LOOP('',(#27775,#27776,#27777,#27778,#27779));
#7610=EDGE_LOOP('',(#27780));
#7611=EDGE_LOOP('',(#27781,#27782,#27783,#27784));
#7612=EDGE_LOOP('',(#27785,#27786,#27787,#27788));
#7613=EDGE_LOOP('',(#27789,#27790,#27791,#27792,#27793,#27794,#27795,#27796,
#27797,#27798,#27799,#27800,#27801,#27802,#27803,#27804,#27805,#27806,#27807,
#27808,#27809,#27810,#27811,#27812,#27813,#27814,#27815,#27816,#27817,#27818,
#27819,#27820,#27821,#27822,#27823,#27824,#27825,#27826,#27827,#27828,#27829,
#27830,#27831,#27832,#27833,#27834,#27835,#27836,#27837,#27838,#27839,#27840,
#27841,#27842,#27843,#27844,#27845,#27846,#27847,#27848,#27849,#27850,#27851,
#27852,#27853,#27854,#27855,#27856,#27857,#27858,#27859,#27860,#27861,#27862,
#27863,#27864,#27865,#27866,#27867,#27868,#27869,#27870,#27871,#27872,#27873,
#27874,#27875,#27876,#27877,#27878,#27879,#27880,#27881,#27882,#27883,#27884,
#27885,#27886,#27887,#27888,#27889,#27890,#27891,#27892,#27893,#27894,#27895,
#27896,#27897,#27898,#27899,#27900,#27901,#27902,#27903,#27904,#27905,#27906,
#27907,#27908,#27909,#27910,#27911,#27912,#27913,#27914,#27915,#27916,#27917,
#27918,#27919,#27920,#27921,#27922,#27923,#27924,#27925,#27926,#27927,#27928,
#27929,#27930,#27931,#27932,#27933,#27934,#27935,#27936,#27937,#27938,#27939,
#27940,#27941,#27942,#27943,#27944,#27945,#27946,#27947,#27948));
#7614=EDGE_LOOP('',(#27949));
#7615=EDGE_LOOP('',(#27950,#27951,#27952,#27953));
#7616=EDGE_LOOP('',(#27954,#27955,#27956,#27957));
#7617=EDGE_LOOP('',(#27958,#27959,#27960,#27961));
#7618=EDGE_LOOP('',(#27962,#27963,#27964,#27965));
#7619=EDGE_LOOP('',(#27966,#27967,#27968,#27969));
#7620=EDGE_LOOP('',(#27970,#27971,#27972,#27973));
#7621=EDGE_LOOP('',(#27974,#27975,#27976,#27977));
#7622=EDGE_LOOP('',(#27978,#27979,#27980,#27981));
#7623=EDGE_LOOP('',(#27982,#27983,#27984,#27985));
#7624=EDGE_LOOP('',(#27986,#27987,#27988,#27989));
#7625=EDGE_LOOP('',(#27990,#27991,#27992,#27993));
#7626=EDGE_LOOP('',(#27994,#27995,#27996,#27997));
#7627=EDGE_LOOP('',(#27998,#27999,#28000,#28001));
#7628=EDGE_LOOP('',(#28002,#28003,#28004,#28005));
#7629=EDGE_LOOP('',(#28006,#28007,#28008,#28009));
#7630=EDGE_LOOP('',(#28010,#28011,#28012,#28013));
#7631=EDGE_LOOP('',(#28014,#28015,#28016,#28017));
#7632=EDGE_LOOP('',(#28018,#28019,#28020,#28021));
#7633=EDGE_LOOP('',(#28022,#28023,#28024,#28025));
#7634=EDGE_LOOP('',(#28026,#28027,#28028,#28029));
#7635=EDGE_LOOP('',(#28030,#28031,#28032,#28033));
#7636=EDGE_LOOP('',(#28034,#28035,#28036,#28037));
#7637=EDGE_LOOP('',(#28038,#28039,#28040,#28041));
#7638=EDGE_LOOP('',(#28042,#28043,#28044,#28045));
#7639=EDGE_LOOP('',(#28046,#28047,#28048,#28049));
#7640=EDGE_LOOP('',(#28050,#28051,#28052,#28053));
#7641=EDGE_LOOP('',(#28054,#28055,#28056,#28057));
#7642=EDGE_LOOP('',(#28058,#28059,#28060,#28061));
#7643=EDGE_LOOP('',(#28062,#28063,#28064,#28065));
#7644=EDGE_LOOP('',(#28066,#28067,#28068,#28069));
#7645=EDGE_LOOP('',(#28070,#28071,#28072,#28073));
#7646=EDGE_LOOP('',(#28074,#28075,#28076,#28077));
#7647=EDGE_LOOP('',(#28078,#28079,#28080,#28081));
#7648=EDGE_LOOP('',(#28082,#28083,#28084,#28085));
#7649=EDGE_LOOP('',(#28086,#28087,#28088,#28089));
#7650=EDGE_LOOP('',(#28090,#28091,#28092,#28093));
#7651=EDGE_LOOP('',(#28094,#28095,#28096,#28097));
#7652=EDGE_LOOP('',(#28098,#28099,#28100,#28101));
#7653=EDGE_LOOP('',(#28102,#28103,#28104,#28105));
#7654=EDGE_LOOP('',(#28106,#28107,#28108,#28109));
#7655=EDGE_LOOP('',(#28110,#28111,#28112,#28113));
#7656=EDGE_LOOP('',(#28114,#28115,#28116,#28117));
#7657=EDGE_LOOP('',(#28118,#28119,#28120,#28121));
#7658=EDGE_LOOP('',(#28122,#28123,#28124,#28125));
#7659=EDGE_LOOP('',(#28126,#28127,#28128,#28129));
#7660=EDGE_LOOP('',(#28130,#28131,#28132,#28133));
#7661=EDGE_LOOP('',(#28134,#28135,#28136,#28137));
#7662=EDGE_LOOP('',(#28138,#28139,#28140,#28141));
#7663=EDGE_LOOP('',(#28142,#28143,#28144,#28145));
#7664=EDGE_LOOP('',(#28146,#28147,#28148,#28149));
#7665=EDGE_LOOP('',(#28150,#28151,#28152,#28153));
#7666=EDGE_LOOP('',(#28154,#28155,#28156,#28157));
#7667=EDGE_LOOP('',(#28158,#28159,#28160,#28161));
#7668=EDGE_LOOP('',(#28162,#28163,#28164,#28165));
#7669=EDGE_LOOP('',(#28166,#28167,#28168,#28169));
#7670=EDGE_LOOP('',(#28170,#28171,#28172,#28173));
#7671=EDGE_LOOP('',(#28174,#28175,#28176,#28177));
#7672=EDGE_LOOP('',(#28178,#28179,#28180,#28181));
#7673=EDGE_LOOP('',(#28182,#28183,#28184,#28185));
#7674=EDGE_LOOP('',(#28186,#28187,#28188,#28189));
#7675=EDGE_LOOP('',(#28190,#28191,#28192,#28193));
#7676=EDGE_LOOP('',(#28194,#28195,#28196,#28197));
#7677=EDGE_LOOP('',(#28198,#28199,#28200,#28201));
#7678=EDGE_LOOP('',(#28202,#28203,#28204,#28205));
#7679=EDGE_LOOP('',(#28206,#28207,#28208,#28209));
#7680=EDGE_LOOP('',(#28210,#28211,#28212,#28213));
#7681=EDGE_LOOP('',(#28214,#28215,#28216,#28217));
#7682=EDGE_LOOP('',(#28218,#28219,#28220,#28221));
#7683=EDGE_LOOP('',(#28222,#28223,#28224,#28225));
#7684=EDGE_LOOP('',(#28226,#28227,#28228,#28229));
#7685=EDGE_LOOP('',(#28230,#28231,#28232,#28233));
#7686=EDGE_LOOP('',(#28234,#28235,#28236,#28237));
#7687=EDGE_LOOP('',(#28238,#28239,#28240,#28241));
#7688=EDGE_LOOP('',(#28242,#28243,#28244,#28245));
#7689=EDGE_LOOP('',(#28246,#28247,#28248,#28249));
#7690=EDGE_LOOP('',(#28250,#28251,#28252,#28253));
#7691=EDGE_LOOP('',(#28254,#28255,#28256,#28257));
#7692=EDGE_LOOP('',(#28258,#28259,#28260,#28261));
#7693=EDGE_LOOP('',(#28262,#28263,#28264,#28265));
#7694=EDGE_LOOP('',(#28266,#28267,#28268,#28269));
#7695=EDGE_LOOP('',(#28270,#28271,#28272,#28273));
#7696=EDGE_LOOP('',(#28274,#28275,#28276,#28277));
#7697=EDGE_LOOP('',(#28278,#28279,#28280,#28281));
#7698=EDGE_LOOP('',(#28282,#28283,#28284,#28285));
#7699=EDGE_LOOP('',(#28286,#28287,#28288,#28289));
#7700=EDGE_LOOP('',(#28290,#28291,#28292,#28293));
#7701=EDGE_LOOP('',(#28294,#28295,#28296,#28297));
#7702=EDGE_LOOP('',(#28298,#28299,#28300,#28301));
#7703=EDGE_LOOP('',(#28302,#28303,#28304,#28305));
#7704=EDGE_LOOP('',(#28306,#28307,#28308,#28309));
#7705=EDGE_LOOP('',(#28310,#28311,#28312,#28313));
#7706=EDGE_LOOP('',(#28314,#28315,#28316,#28317));
#7707=EDGE_LOOP('',(#28318,#28319,#28320,#28321));
#7708=EDGE_LOOP('',(#28322,#28323,#28324,#28325));
#7709=EDGE_LOOP('',(#28326,#28327,#28328,#28329));
#7710=EDGE_LOOP('',(#28330,#28331,#28332,#28333));
#7711=EDGE_LOOP('',(#28334,#28335,#28336,#28337));
#7712=EDGE_LOOP('',(#28338,#28339,#28340,#28341));
#7713=EDGE_LOOP('',(#28342,#28343,#28344,#28345));
#7714=EDGE_LOOP('',(#28346,#28347,#28348,#28349));
#7715=EDGE_LOOP('',(#28350,#28351,#28352,#28353));
#7716=EDGE_LOOP('',(#28354,#28355,#28356,#28357));
#7717=EDGE_LOOP('',(#28358,#28359,#28360,#28361));
#7718=EDGE_LOOP('',(#28362,#28363,#28364,#28365));
#7719=EDGE_LOOP('',(#28366,#28367,#28368,#28369));
#7720=EDGE_LOOP('',(#28370,#28371,#28372,#28373));
#7721=EDGE_LOOP('',(#28374,#28375,#28376,#28377));
#7722=EDGE_LOOP('',(#28378,#28379,#28380,#28381));
#7723=EDGE_LOOP('',(#28382,#28383,#28384,#28385));
#7724=EDGE_LOOP('',(#28386,#28387,#28388,#28389));
#7725=EDGE_LOOP('',(#28390,#28391,#28392,#28393));
#7726=EDGE_LOOP('',(#28394,#28395,#28396,#28397));
#7727=EDGE_LOOP('',(#28398,#28399,#28400,#28401));
#7728=EDGE_LOOP('',(#28402,#28403,#28404,#28405));
#7729=EDGE_LOOP('',(#28406,#28407,#28408,#28409));
#7730=EDGE_LOOP('',(#28410,#28411,#28412,#28413));
#7731=EDGE_LOOP('',(#28414,#28415,#28416,#28417));
#7732=EDGE_LOOP('',(#28418,#28419,#28420,#28421));
#7733=EDGE_LOOP('',(#28422,#28423,#28424,#28425));
#7734=EDGE_LOOP('',(#28426,#28427,#28428,#28429));
#7735=EDGE_LOOP('',(#28430,#28431,#28432,#28433));
#7736=EDGE_LOOP('',(#28434,#28435,#28436,#28437));
#7737=EDGE_LOOP('',(#28438,#28439,#28440,#28441));
#7738=EDGE_LOOP('',(#28442,#28443,#28444,#28445));
#7739=EDGE_LOOP('',(#28446,#28447,#28448,#28449));
#7740=EDGE_LOOP('',(#28450,#28451,#28452,#28453));
#7741=EDGE_LOOP('',(#28454,#28455,#28456,#28457));
#7742=EDGE_LOOP('',(#28458,#28459,#28460,#28461));
#7743=EDGE_LOOP('',(#28462,#28463,#28464,#28465));
#7744=EDGE_LOOP('',(#28466,#28467,#28468,#28469));
#7745=EDGE_LOOP('',(#28470,#28471,#28472,#28473));
#7746=EDGE_LOOP('',(#28474,#28475,#28476,#28477));
#7747=EDGE_LOOP('',(#28478,#28479,#28480,#28481));
#7748=EDGE_LOOP('',(#28482,#28483,#28484,#28485));
#7749=EDGE_LOOP('',(#28486,#28487,#28488,#28489));
#7750=EDGE_LOOP('',(#28490,#28491,#28492,#28493));
#7751=EDGE_LOOP('',(#28494,#28495,#28496,#28497));
#7752=EDGE_LOOP('',(#28498,#28499,#28500,#28501));
#7753=EDGE_LOOP('',(#28502,#28503,#28504,#28505));
#7754=EDGE_LOOP('',(#28506,#28507,#28508,#28509));
#7755=EDGE_LOOP('',(#28510,#28511,#28512,#28513));
#7756=EDGE_LOOP('',(#28514,#28515,#28516,#28517));
#7757=EDGE_LOOP('',(#28518,#28519,#28520,#28521));
#7758=EDGE_LOOP('',(#28522,#28523,#28524,#28525));
#7759=EDGE_LOOP('',(#28526,#28527,#28528,#28529));
#7760=EDGE_LOOP('',(#28530,#28531,#28532,#28533));
#7761=EDGE_LOOP('',(#28534,#28535,#28536,#28537));
#7762=EDGE_LOOP('',(#28538,#28539,#28540,#28541));
#7763=EDGE_LOOP('',(#28542,#28543,#28544,#28545));
#7764=EDGE_LOOP('',(#28546,#28547,#28548,#28549));
#7765=EDGE_LOOP('',(#28550,#28551,#28552,#28553));
#7766=EDGE_LOOP('',(#28554,#28555,#28556,#28557));
#7767=EDGE_LOOP('',(#28558,#28559,#28560,#28561));
#7768=EDGE_LOOP('',(#28562,#28563,#28564,#28565));
#7769=EDGE_LOOP('',(#28566,#28567,#28568,#28569));
#7770=EDGE_LOOP('',(#28570,#28571,#28572,#28573));
#7771=EDGE_LOOP('',(#28574,#28575,#28576,#28577));
#7772=EDGE_LOOP('',(#28578,#28579,#28580,#28581));
#7773=EDGE_LOOP('',(#28582,#28583,#28584,#28585));
#7774=EDGE_LOOP('',(#28586,#28587,#28588,#28589));
#7775=EDGE_LOOP('',(#28590,#28591,#28592,#28593));
#7776=EDGE_LOOP('',(#28594,#28595,#28596,#28597));
#7777=EDGE_LOOP('',(#28598,#28599,#28600,#28601));
#7778=EDGE_LOOP('',(#28602,#28603,#28604,#28605));
#7779=EDGE_LOOP('',(#28606,#28607,#28608,#28609,#28610,#28611,#28612,#28613,
#28614,#28615,#28616,#28617,#28618,#28619,#28620,#28621,#28622,#28623,#28624,
#28625,#28626,#28627,#28628,#28629,#28630,#28631,#28632,#28633,#28634,#28635,
#28636,#28637,#28638,#28639,#28640,#28641,#28642,#28643,#28644,#28645,#28646,
#28647,#28648,#28649,#28650,#28651,#28652,#28653,#28654,#28655,#28656,#28657,
#28658,#28659,#28660,#28661,#28662,#28663,#28664,#28665,#28666,#28667,#28668,
#28669,#28670,#28671,#28672,#28673,#28674,#28675,#28676,#28677,#28678,#28679,
#28680,#28681,#28682,#28683,#28684,#28685,#28686,#28687,#28688,#28689,#28690,
#28691,#28692,#28693,#28694,#28695,#28696,#28697,#28698,#28699,#28700,#28701,
#28702,#28703,#28704,#28705,#28706,#28707,#28708,#28709,#28710,#28711,#28712,
#28713,#28714,#28715,#28716,#28717,#28718,#28719,#28720,#28721,#28722,#28723,
#28724,#28725,#28726,#28727,#28728,#28729,#28730,#28731,#28732,#28733,#28734,
#28735,#28736,#28737,#28738,#28739,#28740,#28741,#28742,#28743,#28744,#28745,
#28746,#28747,#28748,#28749,#28750,#28751,#28752,#28753,#28754,#28755,#28756,
#28757,#28758,#28759,#28760,#28761,#28762,#28763,#28764,#28765));
#7780=EDGE_LOOP('',(#28766,#28767,#28768,#28769));
#10029=LINE('',#57611,#12576);
#10030=LINE('',#57616,#12577);
#10031=LINE('',#57618,#12578);
#10032=LINE('',#57620,#12579);
#10033=LINE('',#57950,#12580);
#10034=LINE('',#57951,#12581);
#10035=LINE('',#57952,#12582);
#10036=LINE('',#57955,#12583);
#10037=LINE('',#57956,#12584);
#10038=LINE('',#57960,#12585);
#10039=LINE('',#57962,#12586);
#10040=LINE('',#57965,#12587);
#10041=LINE('',#57968,#12588);
#10042=LINE('',#57972,#12589);
#10043=LINE('',#57975,#12590);
#10044=LINE('',#57979,#12591);
#10045=LINE('',#57982,#12592);
#10046=LINE('',#57986,#12593);
#10047=LINE('',#57989,#12594);
#10048=LINE('',#57993,#12595);
#10049=LINE('',#57996,#12596);
#10050=LINE('',#58000,#12597);
#10051=LINE('',#58003,#12598);
#10052=LINE('',#58007,#12599);
#10053=LINE('',#58010,#12600);
#10054=LINE('',#58014,#12601);
#10055=LINE('',#58017,#12602);
#10056=LINE('',#58021,#12603);
#10057=LINE('',#58024,#12604);
#10058=LINE('',#58028,#12605);
#10059=LINE('',#58031,#12606);
#10060=LINE('',#58035,#12607);
#10061=LINE('',#58038,#12608);
#10062=LINE('',#58042,#12609);
#10063=LINE('',#58045,#12610);
#10064=LINE('',#58049,#12611);
#10065=LINE('',#58052,#12612);
#10066=LINE('',#58056,#12613);
#10067=LINE('',#58059,#12614);
#10068=LINE('',#58063,#12615);
#10069=LINE('',#58066,#12616);
#10070=LINE('',#58070,#12617);
#10071=LINE('',#58073,#12618);
#10072=LINE('',#58077,#12619);
#10073=LINE('',#58080,#12620);
#10074=LINE('',#58084,#12621);
#10075=LINE('',#58087,#12622);
#10076=LINE('',#58091,#12623);
#10077=LINE('',#58094,#12624);
#10078=LINE('',#58098,#12625);
#10079=LINE('',#58101,#12626);
#10080=LINE('',#58105,#12627);
#10081=LINE('',#58108,#12628);
#10082=LINE('',#58112,#12629);
#10083=LINE('',#58115,#12630);
#10084=LINE('',#58119,#12631);
#10085=LINE('',#58122,#12632);
#10086=LINE('',#58126,#12633);
#10087=LINE('',#58129,#12634);
#10088=LINE('',#58133,#12635);
#10089=LINE('',#58136,#12636);
#10090=LINE('',#58140,#12637);
#10091=LINE('',#58143,#12638);
#10092=LINE('',#58147,#12639);
#10093=LINE('',#58150,#12640);
#10094=LINE('',#58154,#12641);
#10095=LINE('',#58157,#12642);
#10096=LINE('',#58161,#12643);
#10097=LINE('',#58164,#12644);
#10098=LINE('',#58168,#12645);
#10099=LINE('',#58171,#12646);
#10100=LINE('',#58175,#12647);
#10101=LINE('',#58178,#12648);
#10102=LINE('',#58182,#12649);
#10103=LINE('',#58185,#12650);
#10104=LINE('',#58189,#12651);
#10105=LINE('',#58192,#12652);
#10106=LINE('',#58196,#12653);
#10107=LINE('',#58199,#12654);
#10108=LINE('',#58203,#12655);
#10109=LINE('',#58206,#12656);
#10110=LINE('',#58210,#12657);
#10111=LINE('',#58213,#12658);
#10112=LINE('',#58217,#12659);
#10113=LINE('',#58220,#12660);
#10114=LINE('',#58224,#12661);
#10115=LINE('',#58227,#12662);
#10116=LINE('',#58231,#12663);
#10117=LINE('',#58234,#12664);
#10118=LINE('',#58238,#12665);
#10119=LINE('',#58241,#12666);
#10120=LINE('',#58245,#12667);
#10121=LINE('',#58248,#12668);
#10122=LINE('',#58252,#12669);
#10123=LINE('',#58255,#12670);
#10124=LINE('',#58259,#12671);
#10125=LINE('',#58262,#12672);
#10126=LINE('',#58266,#12673);
#10127=LINE('',#58269,#12674);
#10128=LINE('',#58273,#12675);
#10129=LINE('',#58276,#12676);
#10130=LINE('',#58280,#12677);
#10131=LINE('',#58283,#12678);
#10132=LINE('',#58287,#12679);
#10133=LINE('',#58290,#12680);
#10134=LINE('',#58294,#12681);
#10135=LINE('',#58297,#12682);
#10136=LINE('',#58301,#12683);
#10137=LINE('',#58304,#12684);
#10138=LINE('',#58308,#12685);
#10139=LINE('',#58311,#12686);
#10140=LINE('',#58315,#12687);
#10141=LINE('',#58318,#12688);
#10142=LINE('',#58322,#12689);
#10143=LINE('',#58325,#12690);
#10144=LINE('',#58329,#12691);
#10145=LINE('',#58332,#12692);
#10146=LINE('',#58336,#12693);
#10147=LINE('',#58339,#12694);
#10148=LINE('',#58343,#12695);
#10149=LINE('',#58346,#12696);
#10150=LINE('',#58350,#12697);
#10151=LINE('',#58353,#12698);
#10152=LINE('',#58357,#12699);
#10153=LINE('',#58360,#12700);
#10154=LINE('',#58364,#12701);
#10155=LINE('',#58367,#12702);
#10156=LINE('',#58371,#12703);
#10157=LINE('',#58374,#12704);
#10158=LINE('',#58378,#12705);
#10159=LINE('',#58381,#12706);
#10160=LINE('',#58385,#12707);
#10161=LINE('',#58388,#12708);
#10162=LINE('',#58392,#12709);
#10163=LINE('',#58395,#12710);
#10164=LINE('',#58399,#12711);
#10165=LINE('',#58402,#12712);
#10166=LINE('',#58406,#12713);
#10167=LINE('',#58409,#12714);
#10168=LINE('',#58413,#12715);
#10169=LINE('',#58416,#12716);
#10170=LINE('',#58420,#12717);
#10171=LINE('',#58423,#12718);
#10172=LINE('',#58427,#12719);
#10173=LINE('',#58430,#12720);
#10174=LINE('',#58434,#12721);
#10175=LINE('',#58437,#12722);
#10176=LINE('',#58441,#12723);
#10177=LINE('',#58444,#12724);
#10178=LINE('',#58448,#12725);
#10179=LINE('',#58451,#12726);
#10180=LINE('',#58455,#12727);
#10181=LINE('',#58458,#12728);
#10182=LINE('',#58462,#12729);
#10183=LINE('',#58465,#12730);
#10184=LINE('',#58469,#12731);
#10185=LINE('',#58472,#12732);
#10186=LINE('',#58476,#12733);
#10187=LINE('',#58479,#12734);
#10188=LINE('',#58483,#12735);
#10189=LINE('',#58486,#12736);
#10190=LINE('',#58490,#12737);
#10191=LINE('',#58493,#12738);
#10192=LINE('',#58497,#12739);
#10193=LINE('',#58500,#12740);
#10194=LINE('',#58504,#12741);
#10195=LINE('',#58507,#12742);
#10196=LINE('',#58512,#12743);
#10197=LINE('',#58591,#12744);
#10198=LINE('',#58594,#12745);
#10199=LINE('',#58598,#12746);
#12576=VECTOR('',#45127,30.);
#12577=VECTOR('',#45132,10.);
#12578=VECTOR('',#45133,10.);
#12579=VECTOR('',#45134,10.);
#12580=VECTOR('',#45467,10.);
#12581=VECTOR('',#45468,10.);
#12582=VECTOR('',#45469,10.);
#12583=VECTOR('',#45472,10.);
#12584=VECTOR('',#45473,10.);
#12585=VECTOR('',#45478,10.);
#12586=VECTOR('',#45481,10.);
#12587=VECTOR('',#45484,10.);
#12588=VECTOR('',#45487,10.);
#12589=VECTOR('',#45492,10.);
#12590=VECTOR('',#45495,10.);
#12591=VECTOR('',#45500,10.);
#12592=VECTOR('',#45503,10.);
#12593=VECTOR('',#45508,10.);
#12594=VECTOR('',#45511,10.);
#12595=VECTOR('',#45516,10.);
#12596=VECTOR('',#45519,10.);
#12597=VECTOR('',#45524,10.);
#12598=VECTOR('',#45527,10.);
#12599=VECTOR('',#45532,10.);
#12600=VECTOR('',#45535,10.);
#12601=VECTOR('',#45540,10.);
#12602=VECTOR('',#45543,10.);
#12603=VECTOR('',#45548,10.);
#12604=VECTOR('',#45551,10.);
#12605=VECTOR('',#45556,10.);
#12606=VECTOR('',#45559,10.);
#12607=VECTOR('',#45564,10.);
#12608=VECTOR('',#45567,10.);
#12609=VECTOR('',#45572,10.);
#12610=VECTOR('',#45575,10.);
#12611=VECTOR('',#45580,10.);
#12612=VECTOR('',#45583,10.);
#12613=VECTOR('',#45588,10.);
#12614=VECTOR('',#45591,10.);
#12615=VECTOR('',#45596,10.);
#12616=VECTOR('',#45599,10.);
#12617=VECTOR('',#45604,10.);
#12618=VECTOR('',#45607,10.);
#12619=VECTOR('',#45612,10.);
#12620=VECTOR('',#45615,10.);
#12621=VECTOR('',#45620,10.);
#12622=VECTOR('',#45623,10.);
#12623=VECTOR('',#45628,10.);
#12624=VECTOR('',#45631,10.);
#12625=VECTOR('',#45636,10.);
#12626=VECTOR('',#45639,10.);
#12627=VECTOR('',#45644,10.);
#12628=VECTOR('',#45647,10.);
#12629=VECTOR('',#45652,10.);
#12630=VECTOR('',#45655,10.);
#12631=VECTOR('',#45660,10.);
#12632=VECTOR('',#45663,10.);
#12633=VECTOR('',#45668,10.);
#12634=VECTOR('',#45671,10.);
#12635=VECTOR('',#45676,10.);
#12636=VECTOR('',#45679,10.);
#12637=VECTOR('',#45684,10.);
#12638=VECTOR('',#45687,10.);
#12639=VECTOR('',#45692,10.);
#12640=VECTOR('',#45695,10.);
#12641=VECTOR('',#45700,10.);
#12642=VECTOR('',#45703,10.);
#12643=VECTOR('',#45708,10.);
#12644=VECTOR('',#45711,10.);
#12645=VECTOR('',#45716,10.);
#12646=VECTOR('',#45719,10.);
#12647=VECTOR('',#45724,10.);
#12648=VECTOR('',#45727,10.);
#12649=VECTOR('',#45732,10.);
#12650=VECTOR('',#45735,10.);
#12651=VECTOR('',#45740,10.);
#12652=VECTOR('',#45743,10.);
#12653=VECTOR('',#45748,10.);
#12654=VECTOR('',#45751,10.);
#12655=VECTOR('',#45756,10.);
#12656=VECTOR('',#45759,10.);
#12657=VECTOR('',#45764,10.);
#12658=VECTOR('',#45767,10.);
#12659=VECTOR('',#45772,10.);
#12660=VECTOR('',#45775,10.);
#12661=VECTOR('',#45780,10.);
#12662=VECTOR('',#45783,10.);
#12663=VECTOR('',#45788,10.);
#12664=VECTOR('',#45791,10.);
#12665=VECTOR('',#45796,10.);
#12666=VECTOR('',#45799,10.);
#12667=VECTOR('',#45804,10.);
#12668=VECTOR('',#45807,10.);
#12669=VECTOR('',#45812,10.);
#12670=VECTOR('',#45815,10.);
#12671=VECTOR('',#45820,10.);
#12672=VECTOR('',#45823,10.);
#12673=VECTOR('',#45828,10.);
#12674=VECTOR('',#45831,10.);
#12675=VECTOR('',#45836,10.);
#12676=VECTOR('',#45839,10.);
#12677=VECTOR('',#45844,10.);
#12678=VECTOR('',#45847,10.);
#12679=VECTOR('',#45852,10.);
#12680=VECTOR('',#45855,10.);
#12681=VECTOR('',#45860,10.);
#12682=VECTOR('',#45863,10.);
#12683=VECTOR('',#45868,10.);
#12684=VECTOR('',#45871,10.);
#12685=VECTOR('',#45876,10.);
#12686=VECTOR('',#45879,10.);
#12687=VECTOR('',#45884,10.);
#12688=VECTOR('',#45887,10.);
#12689=VECTOR('',#45892,10.);
#12690=VECTOR('',#45895,10.);
#12691=VECTOR('',#45900,10.);
#12692=VECTOR('',#45903,10.);
#12693=VECTOR('',#45908,10.);
#12694=VECTOR('',#45911,10.);
#12695=VECTOR('',#45916,10.);
#12696=VECTOR('',#45919,10.);
#12697=VECTOR('',#45924,10.);
#12698=VECTOR('',#45927,10.);
#12699=VECTOR('',#45932,10.);
#12700=VECTOR('',#45935,10.);
#12701=VECTOR('',#45940,10.);
#12702=VECTOR('',#45943,10.);
#12703=VECTOR('',#45948,10.);
#12704=VECTOR('',#45951,10.);
#12705=VECTOR('',#45956,10.);
#12706=VECTOR('',#45959,10.);
#12707=VECTOR('',#45964,10.);
#12708=VECTOR('',#45967,10.);
#12709=VECTOR('',#45972,10.);
#12710=VECTOR('',#45975,10.);
#12711=VECTOR('',#45980,10.);
#12712=VECTOR('',#45983,10.);
#12713=VECTOR('',#45988,10.);
#12714=VECTOR('',#45991,10.);
#12715=VECTOR('',#45996,10.);
#12716=VECTOR('',#45999,10.);
#12717=VECTOR('',#46004,10.);
#12718=VECTOR('',#46007,10.);
#12719=VECTOR('',#46012,10.);
#12720=VECTOR('',#46015,10.);
#12721=VECTOR('',#46020,10.);
#12722=VECTOR('',#46023,10.);
#12723=VECTOR('',#46028,10.);
#12724=VECTOR('',#46031,10.);
#12725=VECTOR('',#46036,10.);
#12726=VECTOR('',#46039,10.);
#12727=VECTOR('',#46044,10.);
#12728=VECTOR('',#46047,10.);
#12729=VECTOR('',#46052,10.);
#12730=VECTOR('',#46055,10.);
#12731=VECTOR('',#46060,10.);
#12732=VECTOR('',#46063,10.);
#12733=VECTOR('',#46068,10.);
#12734=VECTOR('',#46071,10.);
#12735=VECTOR('',#46076,10.);
#12736=VECTOR('',#46079,10.);
#12737=VECTOR('',#46084,10.);
#12738=VECTOR('',#46087,10.);
#12739=VECTOR('',#46092,10.);
#12740=VECTOR('',#46095,10.);
#12741=VECTOR('',#46100,10.);
#12742=VECTOR('',#46103,10.);
#12743=VECTOR('',#46110,10.);
#12744=VECTOR('',#46265,10.);
#12745=VECTOR('',#46268,10.);
#12746=VECTOR('',#46273,10.);
#15508=VERTEX_POINT('',#57602);
#15509=VERTEX_POINT('',#57604);
#15510=VERTEX_POINT('',#57606);
#15511=VERTEX_POINT('',#57610);
#15512=VERTEX_POINT('',#57614);
#15513=VERTEX_POINT('',#57615);
#15514=VERTEX_POINT('',#57617);
#15515=VERTEX_POINT('',#57619);
#15516=VERTEX_POINT('',#57623);
#15517=VERTEX_POINT('',#57627);
#15518=VERTEX_POINT('',#57628);
#15519=VERTEX_POINT('',#57630);
#15520=VERTEX_POINT('',#57632);
#15521=VERTEX_POINT('',#57634);
#15522=VERTEX_POINT('',#57636);
#15523=VERTEX_POINT('',#57638);
#15524=VERTEX_POINT('',#57640);
#15525=VERTEX_POINT('',#57642);
#15526=VERTEX_POINT('',#57644);
#15527=VERTEX_POINT('',#57646);
#15528=VERTEX_POINT('',#57648);
#15529=VERTEX_POINT('',#57650);
#15530=VERTEX_POINT('',#57652);
#15531=VERTEX_POINT('',#57654);
#15532=VERTEX_POINT('',#57656);
#15533=VERTEX_POINT('',#57658);
#15534=VERTEX_POINT('',#57660);
#15535=VERTEX_POINT('',#57662);
#15536=VERTEX_POINT('',#57664);
#15537=VERTEX_POINT('',#57666);
#15538=VERTEX_POINT('',#57668);
#15539=VERTEX_POINT('',#57670);
#15540=VERTEX_POINT('',#57672);
#15541=VERTEX_POINT('',#57674);
#15542=VERTEX_POINT('',#57676);
#15543=VERTEX_POINT('',#57678);
#15544=VERTEX_POINT('',#57680);
#15545=VERTEX_POINT('',#57682);
#15546=VERTEX_POINT('',#57684);
#15547=VERTEX_POINT('',#57686);
#15548=VERTEX_POINT('',#57688);
#15549=VERTEX_POINT('',#57690);
#15550=VERTEX_POINT('',#57692);
#15551=VERTEX_POINT('',#57694);
#15552=VERTEX_POINT('',#57696);
#15553=VERTEX_POINT('',#57698);
#15554=VERTEX_POINT('',#57700);
#15555=VERTEX_POINT('',#57702);
#15556=VERTEX_POINT('',#57704);
#15557=VERTEX_POINT('',#57706);
#15558=VERTEX_POINT('',#57708);
#15559=VERTEX_POINT('',#57710);
#15560=VERTEX_POINT('',#57712);
#15561=VERTEX_POINT('',#57714);
#15562=VERTEX_POINT('',#57716);
#15563=VERTEX_POINT('',#57718);
#15564=VERTEX_POINT('',#57720);
#15565=VERTEX_POINT('',#57722);
#15566=VERTEX_POINT('',#57724);
#15567=VERTEX_POINT('',#57726);
#15568=VERTEX_POINT('',#57728);
#15569=VERTEX_POINT('',#57730);
#15570=VERTEX_POINT('',#57732);
#15571=VERTEX_POINT('',#57734);
#15572=VERTEX_POINT('',#57736);
#15573=VERTEX_POINT('',#57738);
#15574=VERTEX_POINT('',#57740);
#15575=VERTEX_POINT('',#57742);
#15576=VERTEX_POINT('',#57744);
#15577=VERTEX_POINT('',#57746);
#15578=VERTEX_POINT('',#57748);
#15579=VERTEX_POINT('',#57750);
#15580=VERTEX_POINT('',#57752);
#15581=VERTEX_POINT('',#57754);
#15582=VERTEX_POINT('',#57756);
#15583=VERTEX_POINT('',#57758);
#15584=VERTEX_POINT('',#57760);
#15585=VERTEX_POINT('',#57762);
#15586=VERTEX_POINT('',#57764);
#15587=VERTEX_POINT('',#57766);
#15588=VERTEX_POINT('',#57768);
#15589=VERTEX_POINT('',#57770);
#15590=VERTEX_POINT('',#57772);
#15591=VERTEX_POINT('',#57774);
#15592=VERTEX_POINT('',#57776);
#15593=VERTEX_POINT('',#57778);
#15594=VERTEX_POINT('',#57780);
#15595=VERTEX_POINT('',#57782);
#15596=VERTEX_POINT('',#57784);
#15597=VERTEX_POINT('',#57786);
#15598=VERTEX_POINT('',#57788);
#15599=VERTEX_POINT('',#57790);
#15600=VERTEX_POINT('',#57792);
#15601=VERTEX_POINT('',#57794);
#15602=VERTEX_POINT('',#57796);
#15603=VERTEX_POINT('',#57798);
#15604=VERTEX_POINT('',#57800);
#15605=VERTEX_POINT('',#57802);
#15606=VERTEX_POINT('',#57804);
#15607=VERTEX_POINT('',#57806);
#15608=VERTEX_POINT('',#57808);
#15609=VERTEX_POINT('',#57810);
#15610=VERTEX_POINT('',#57812);
#15611=VERTEX_POINT('',#57814);
#15612=VERTEX_POINT('',#57816);
#15613=VERTEX_POINT('',#57818);
#15614=VERTEX_POINT('',#57820);
#15615=VERTEX_POINT('',#57822);
#15616=VERTEX_POINT('',#57824);
#15617=VERTEX_POINT('',#57826);
#15618=VERTEX_POINT('',#57828);
#15619=VERTEX_POINT('',#57830);
#15620=VERTEX_POINT('',#57832);
#15621=VERTEX_POINT('',#57834);
#15622=VERTEX_POINT('',#57836);
#15623=VERTEX_POINT('',#57838);
#15624=VERTEX_POINT('',#57840);
#15625=VERTEX_POINT('',#57842);
#15626=VERTEX_POINT('',#57844);
#15627=VERTEX_POINT('',#57846);
#15628=VERTEX_POINT('',#57848);
#15629=VERTEX_POINT('',#57850);
#15630=VERTEX_POINT('',#57852);
#15631=VERTEX_POINT('',#57854);
#15632=VERTEX_POINT('',#57856);
#15633=VERTEX_POINT('',#57858);
#15634=VERTEX_POINT('',#57860);
#15635=VERTEX_POINT('',#57862);
#15636=VERTEX_POINT('',#57864);
#15637=VERTEX_POINT('',#57866);
#15638=VERTEX_POINT('',#57868);
#15639=VERTEX_POINT('',#57870);
#15640=VERTEX_POINT('',#57872);
#15641=VERTEX_POINT('',#57874);
#15642=VERTEX_POINT('',#57876);
#15643=VERTEX_POINT('',#57878);
#15644=VERTEX_POINT('',#57880);
#15645=VERTEX_POINT('',#57882);
#15646=VERTEX_POINT('',#57884);
#15647=VERTEX_POINT('',#57886);
#15648=VERTEX_POINT('',#57888);
#15649=VERTEX_POINT('',#57890);
#15650=VERTEX_POINT('',#57892);
#15651=VERTEX_POINT('',#57894);
#15652=VERTEX_POINT('',#57896);
#15653=VERTEX_POINT('',#57898);
#15654=VERTEX_POINT('',#57900);
#15655=VERTEX_POINT('',#57902);
#15656=VERTEX_POINT('',#57904);
#15657=VERTEX_POINT('',#57906);
#15658=VERTEX_POINT('',#57908);
#15659=VERTEX_POINT('',#57910);
#15660=VERTEX_POINT('',#57912);
#15661=VERTEX_POINT('',#57914);
#15662=VERTEX_POINT('',#57916);
#15663=VERTEX_POINT('',#57918);
#15664=VERTEX_POINT('',#57920);
#15665=VERTEX_POINT('',#57922);
#15666=VERTEX_POINT('',#57924);
#15667=VERTEX_POINT('',#57926);
#15668=VERTEX_POINT('',#57928);
#15669=VERTEX_POINT('',#57930);
#15670=VERTEX_POINT('',#57932);
#15671=VERTEX_POINT('',#57934);
#15672=VERTEX_POINT('',#57936);
#15673=VERTEX_POINT('',#57938);
#15674=VERTEX_POINT('',#57940);
#15675=VERTEX_POINT('',#57942);
#15676=VERTEX_POINT('',#57944);
#15677=VERTEX_POINT('',#57948);
#15678=VERTEX_POINT('',#57949);
#15679=VERTEX_POINT('',#57954);
#15680=VERTEX_POINT('',#57958);
#15681=VERTEX_POINT('',#57964);
#15682=VERTEX_POINT('',#57966);
#15683=VERTEX_POINT('',#57970);
#15684=VERTEX_POINT('',#57974);
#15685=VERTEX_POINT('',#57978);
#15686=VERTEX_POINT('',#57980);
#15687=VERTEX_POINT('',#57984);
#15688=VERTEX_POINT('',#57988);
#15689=VERTEX_POINT('',#57992);
#15690=VERTEX_POINT('',#57994);
#15691=VERTEX_POINT('',#57998);
#15692=VERTEX_POINT('',#58002);
#15693=VERTEX_POINT('',#58006);
#15694=VERTEX_POINT('',#58008);
#15695=VERTEX_POINT('',#58012);
#15696=VERTEX_POINT('',#58016);
#15697=VERTEX_POINT('',#58020);
#15698=VERTEX_POINT('',#58022);
#15699=VERTEX_POINT('',#58026);
#15700=VERTEX_POINT('',#58030);
#15701=VERTEX_POINT('',#58034);
#15702=VERTEX_POINT('',#58036);
#15703=VERTEX_POINT('',#58040);
#15704=VERTEX_POINT('',#58044);
#15705=VERTEX_POINT('',#58048);
#15706=VERTEX_POINT('',#58050);
#15707=VERTEX_POINT('',#58054);
#15708=VERTEX_POINT('',#58058);
#15709=VERTEX_POINT('',#58062);
#15710=VERTEX_POINT('',#58064);
#15711=VERTEX_POINT('',#58068);
#15712=VERTEX_POINT('',#58072);
#15713=VERTEX_POINT('',#58076);
#15714=VERTEX_POINT('',#58078);
#15715=VERTEX_POINT('',#58082);
#15716=VERTEX_POINT('',#58086);
#15717=VERTEX_POINT('',#58090);
#15718=VERTEX_POINT('',#58092);
#15719=VERTEX_POINT('',#58096);
#15720=VERTEX_POINT('',#58100);
#15721=VERTEX_POINT('',#58104);
#15722=VERTEX_POINT('',#58106);
#15723=VERTEX_POINT('',#58110);
#15724=VERTEX_POINT('',#58114);
#15725=VERTEX_POINT('',#58118);
#15726=VERTEX_POINT('',#58120);
#15727=VERTEX_POINT('',#58124);
#15728=VERTEX_POINT('',#58128);
#15729=VERTEX_POINT('',#58132);
#15730=VERTEX_POINT('',#58134);
#15731=VERTEX_POINT('',#58138);
#15732=VERTEX_POINT('',#58142);
#15733=VERTEX_POINT('',#58146);
#15734=VERTEX_POINT('',#58148);
#15735=VERTEX_POINT('',#58152);
#15736=VERTEX_POINT('',#58156);
#15737=VERTEX_POINT('',#58160);
#15738=VERTEX_POINT('',#58162);
#15739=VERTEX_POINT('',#58166);
#15740=VERTEX_POINT('',#58170);
#15741=VERTEX_POINT('',#58174);
#15742=VERTEX_POINT('',#58176);
#15743=VERTEX_POINT('',#58180);
#15744=VERTEX_POINT('',#58184);
#15745=VERTEX_POINT('',#58188);
#15746=VERTEX_POINT('',#58190);
#15747=VERTEX_POINT('',#58194);
#15748=VERTEX_POINT('',#58198);
#15749=VERTEX_POINT('',#58202);
#15750=VERTEX_POINT('',#58204);
#15751=VERTEX_POINT('',#58208);
#15752=VERTEX_POINT('',#58212);
#15753=VERTEX_POINT('',#58216);
#15754=VERTEX_POINT('',#58218);
#15755=VERTEX_POINT('',#58222);
#15756=VERTEX_POINT('',#58226);
#15757=VERTEX_POINT('',#58230);
#15758=VERTEX_POINT('',#58232);
#15759=VERTEX_POINT('',#58236);
#15760=VERTEX_POINT('',#58240);
#15761=VERTEX_POINT('',#58244);
#15762=VERTEX_POINT('',#58246);
#15763=VERTEX_POINT('',#58250);
#15764=VERTEX_POINT('',#58254);
#15765=VERTEX_POINT('',#58258);
#15766=VERTEX_POINT('',#58260);
#15767=VERTEX_POINT('',#58264);
#15768=VERTEX_POINT('',#58268);
#15769=VERTEX_POINT('',#58272);
#15770=VERTEX_POINT('',#58274);
#15771=VERTEX_POINT('',#58278);
#15772=VERTEX_POINT('',#58282);
#15773=VERTEX_POINT('',#58286);
#15774=VERTEX_POINT('',#58288);
#15775=VERTEX_POINT('',#58292);
#15776=VERTEX_POINT('',#58296);
#15777=VERTEX_POINT('',#58300);
#15778=VERTEX_POINT('',#58302);
#15779=VERTEX_POINT('',#58306);
#15780=VERTEX_POINT('',#58310);
#15781=VERTEX_POINT('',#58314);
#15782=VERTEX_POINT('',#58316);
#15783=VERTEX_POINT('',#58320);
#15784=VERTEX_POINT('',#58324);
#15785=VERTEX_POINT('',#58328);
#15786=VERTEX_POINT('',#58330);
#15787=VERTEX_POINT('',#58334);
#15788=VERTEX_POINT('',#58338);
#15789=VERTEX_POINT('',#58342);
#15790=VERTEX_POINT('',#58344);
#15791=VERTEX_POINT('',#58348);
#15792=VERTEX_POINT('',#58352);
#15793=VERTEX_POINT('',#58356);
#15794=VERTEX_POINT('',#58358);
#15795=VERTEX_POINT('',#58362);
#15796=VERTEX_POINT('',#58366);
#15797=VERTEX_POINT('',#58370);
#15798=VERTEX_POINT('',#58372);
#15799=VERTEX_POINT('',#58376);
#15800=VERTEX_POINT('',#58380);
#15801=VERTEX_POINT('',#58384);
#15802=VERTEX_POINT('',#58386);
#15803=VERTEX_POINT('',#58390);
#15804=VERTEX_POINT('',#58394);
#15805=VERTEX_POINT('',#58398);
#15806=VERTEX_POINT('',#58400);
#15807=VERTEX_POINT('',#58404);
#15808=VERTEX_POINT('',#58408);
#15809=VERTEX_POINT('',#58412);
#15810=VERTEX_POINT('',#58414);
#15811=VERTEX_POINT('',#58418);
#15812=VERTEX_POINT('',#58422);
#15813=VERTEX_POINT('',#58426);
#15814=VERTEX_POINT('',#58428);
#15815=VERTEX_POINT('',#58432);
#15816=VERTEX_POINT('',#58436);
#15817=VERTEX_POINT('',#58440);
#15818=VERTEX_POINT('',#58442);
#15819=VERTEX_POINT('',#58446);
#15820=VERTEX_POINT('',#58450);
#15821=VERTEX_POINT('',#58454);
#15822=VERTEX_POINT('',#58456);
#15823=VERTEX_POINT('',#58460);
#15824=VERTEX_POINT('',#58464);
#15825=VERTEX_POINT('',#58468);
#15826=VERTEX_POINT('',#58470);
#15827=VERTEX_POINT('',#58474);
#15828=VERTEX_POINT('',#58478);
#15829=VERTEX_POINT('',#58482);
#15830=VERTEX_POINT('',#58484);
#15831=VERTEX_POINT('',#58488);
#15832=VERTEX_POINT('',#58492);
#15833=VERTEX_POINT('',#58496);
#15834=VERTEX_POINT('',#58498);
#15835=VERTEX_POINT('',#58502);
#15836=VERTEX_POINT('',#58506);
#15837=VERTEX_POINT('',#58510);
#15838=VERTEX_POINT('',#58590);
#15839=VERTEX_POINT('',#58592);
#15840=VERTEX_POINT('',#58596);
#19787=EDGE_CURVE('',#15508,#15508,#3518,.T.);
#19788=EDGE_CURVE('',#15508,#15509,#3519,.T.);
#19789=EDGE_CURVE('',#15509,#15510,#3520,.T.);
#19790=EDGE_CURVE('',#15510,#15509,#3521,.T.);
#19791=EDGE_CURVE('',#15510,#15511,#10029,.T.);
#19792=EDGE_CURVE('',#15511,#15511,#3522,.T.);
#19793=EDGE_CURVE('',#15512,#15513,#10030,.T.);
#19794=EDGE_CURVE('',#15513,#15514,#10031,.T.);
#19795=EDGE_CURVE('',#15514,#15515,#10032,.T.);
#19796=EDGE_CURVE('',#15515,#15512,#3523,.T.);
#19797=EDGE_CURVE('',#15516,#15516,#3524,.T.);
#19798=EDGE_CURVE('',#15516,#15511,#3525,.T.);
#19799=EDGE_CURVE('',#15517,#15518,#3526,.T.);
#19800=EDGE_CURVE('',#15518,#15519,#3527,.T.);
#19801=EDGE_CURVE('',#15519,#15520,#3528,.T.);
#19802=EDGE_CURVE('',#15521,#15520,#3529,.T.);
#19803=EDGE_CURVE('',#15521,#15522,#3530,.T.);
#19804=EDGE_CURVE('',#15522,#15523,#3531,.T.);
#19805=EDGE_CURVE('',#15523,#15524,#3532,.T.);
#19806=EDGE_CURVE('',#15525,#15524,#3533,.T.);
#19807=EDGE_CURVE('',#15525,#15526,#3534,.T.);
#19808=EDGE_CURVE('',#15526,#15527,#3535,.T.);
#19809=EDGE_CURVE('',#15527,#15528,#3536,.T.);
#19810=EDGE_CURVE('',#15529,#15528,#3537,.T.);
#19811=EDGE_CURVE('',#15529,#15530,#3538,.T.);
#19812=EDGE_CURVE('',#15530,#15531,#3539,.T.);
#19813=EDGE_CURVE('',#15531,#15532,#3540,.T.);
#19814=EDGE_CURVE('',#15533,#15532,#3541,.T.);
#19815=EDGE_CURVE('',#15533,#15534,#3542,.T.);
#19816=EDGE_CURVE('',#15534,#15535,#3543,.T.);
#19817=EDGE_CURVE('',#15535,#15536,#3544,.T.);
#19818=EDGE_CURVE('',#15537,#15536,#3545,.T.);
#19819=EDGE_CURVE('',#15537,#15538,#3546,.T.);
#19820=EDGE_CURVE('',#15538,#15539,#3547,.T.);
#19821=EDGE_CURVE('',#15539,#15540,#3548,.T.);
#19822=EDGE_CURVE('',#15541,#15540,#3549,.T.);
#19823=EDGE_CURVE('',#15541,#15542,#3550,.T.);
#19824=EDGE_CURVE('',#15542,#15543,#3551,.T.);
#19825=EDGE_CURVE('',#15543,#15544,#3552,.T.);
#19826=EDGE_CURVE('',#15545,#15544,#3553,.T.);
#19827=EDGE_CURVE('',#15545,#15546,#3554,.T.);
#19828=EDGE_CURVE('',#15546,#15547,#3555,.T.);
#19829=EDGE_CURVE('',#15547,#15548,#3556,.T.);
#19830=EDGE_CURVE('',#15549,#15548,#3557,.T.);
#19831=EDGE_CURVE('',#15549,#15550,#3558,.T.);
#19832=EDGE_CURVE('',#15550,#15551,#3559,.T.);
#19833=EDGE_CURVE('',#15551,#15552,#3560,.T.);
#19834=EDGE_CURVE('',#15553,#15552,#3561,.T.);
#19835=EDGE_CURVE('',#15553,#15554,#3562,.T.);
#19836=EDGE_CURVE('',#15554,#15555,#3563,.T.);
#19837=EDGE_CURVE('',#15555,#15556,#3564,.T.);
#19838=EDGE_CURVE('',#15557,#15556,#3565,.T.);
#19839=EDGE_CURVE('',#15557,#15558,#3566,.T.);
#19840=EDGE_CURVE('',#15558,#15559,#3567,.T.);
#19841=EDGE_CURVE('',#15559,#15560,#3568,.T.);
#19842=EDGE_CURVE('',#15561,#15560,#3569,.T.);
#19843=EDGE_CURVE('',#15561,#15562,#3570,.T.);
#19844=EDGE_CURVE('',#15562,#15563,#3571,.T.);
#19845=EDGE_CURVE('',#15563,#15564,#3572,.T.);
#19846=EDGE_CURVE('',#15565,#15564,#3573,.T.);
#19847=EDGE_CURVE('',#15565,#15566,#3574,.T.);
#19848=EDGE_CURVE('',#15566,#15567,#3575,.T.);
#19849=EDGE_CURVE('',#15567,#15568,#3576,.T.);
#19850=EDGE_CURVE('',#15569,#15568,#3577,.T.);
#19851=EDGE_CURVE('',#15569,#15570,#3578,.T.);
#19852=EDGE_CURVE('',#15570,#15571,#3579,.T.);
#19853=EDGE_CURVE('',#15571,#15572,#3580,.T.);
#19854=EDGE_CURVE('',#15573,#15572,#3581,.T.);
#19855=EDGE_CURVE('',#15573,#15574,#3582,.T.);
#19856=EDGE_CURVE('',#15574,#15575,#3583,.T.);
#19857=EDGE_CURVE('',#15575,#15576,#3584,.T.);
#19858=EDGE_CURVE('',#15577,#15576,#3585,.T.);
#19859=EDGE_CURVE('',#15577,#15578,#3586,.T.);
#19860=EDGE_CURVE('',#15578,#15579,#3587,.T.);
#19861=EDGE_CURVE('',#15579,#15580,#3588,.T.);
#19862=EDGE_CURVE('',#15581,#15580,#3589,.T.);
#19863=EDGE_CURVE('',#15581,#15582,#3590,.T.);
#19864=EDGE_CURVE('',#15582,#15583,#3591,.T.);
#19865=EDGE_CURVE('',#15583,#15584,#3592,.T.);
#19866=EDGE_CURVE('',#15585,#15584,#3593,.T.);
#19867=EDGE_CURVE('',#15585,#15586,#3594,.T.);
#19868=EDGE_CURVE('',#15586,#15587,#3595,.T.);
#19869=EDGE_CURVE('',#15587,#15588,#3596,.T.);
#19870=EDGE_CURVE('',#15589,#15588,#3597,.T.);
#19871=EDGE_CURVE('',#15589,#15590,#3598,.T.);
#19872=EDGE_CURVE('',#15590,#15591,#3599,.T.);
#19873=EDGE_CURVE('',#15591,#15592,#3600,.T.);
#19874=EDGE_CURVE('',#15593,#15592,#3601,.T.);
#19875=EDGE_CURVE('',#15593,#15594,#3602,.T.);
#19876=EDGE_CURVE('',#15594,#15595,#3603,.T.);
#19877=EDGE_CURVE('',#15595,#15596,#3604,.T.);
#19878=EDGE_CURVE('',#15597,#15596,#3605,.T.);
#19879=EDGE_CURVE('',#15597,#15598,#3606,.T.);
#19880=EDGE_CURVE('',#15598,#15599,#3607,.T.);
#19881=EDGE_CURVE('',#15599,#15600,#3608,.T.);
#19882=EDGE_CURVE('',#15601,#15600,#3609,.T.);
#19883=EDGE_CURVE('',#15601,#15602,#3610,.T.);
#19884=EDGE_CURVE('',#15602,#15603,#3611,.T.);
#19885=EDGE_CURVE('',#15603,#15604,#3612,.T.);
#19886=EDGE_CURVE('',#15605,#15604,#3613,.T.);
#19887=EDGE_CURVE('',#15605,#15606,#3614,.T.);
#19888=EDGE_CURVE('',#15606,#15607,#3615,.T.);
#19889=EDGE_CURVE('',#15607,#15608,#3616,.T.);
#19890=EDGE_CURVE('',#15609,#15608,#3617,.T.);
#19891=EDGE_CURVE('',#15609,#15610,#3618,.T.);
#19892=EDGE_CURVE('',#15610,#15611,#3619,.T.);
#19893=EDGE_CURVE('',#15611,#15612,#3620,.T.);
#19894=EDGE_CURVE('',#15613,#15612,#3621,.T.);
#19895=EDGE_CURVE('',#15613,#15614,#3622,.T.);
#19896=EDGE_CURVE('',#15614,#15615,#3623,.T.);
#19897=EDGE_CURVE('',#15615,#15616,#3624,.T.);
#19898=EDGE_CURVE('',#15617,#15616,#3625,.T.);
#19899=EDGE_CURVE('',#15617,#15618,#3626,.T.);
#19900=EDGE_CURVE('',#15618,#15619,#3627,.T.);
#19901=EDGE_CURVE('',#15619,#15620,#3628,.T.);
#19902=EDGE_CURVE('',#15621,#15620,#3629,.T.);
#19903=EDGE_CURVE('',#15621,#15622,#3630,.T.);
#19904=EDGE_CURVE('',#15622,#15623,#3631,.T.);
#19905=EDGE_CURVE('',#15623,#15624,#3632,.T.);
#19906=EDGE_CURVE('',#15625,#15624,#3633,.T.);
#19907=EDGE_CURVE('',#15625,#15626,#3634,.T.);
#19908=EDGE_CURVE('',#15626,#15627,#3635,.T.);
#19909=EDGE_CURVE('',#15627,#15628,#3636,.T.);
#19910=EDGE_CURVE('',#15629,#15628,#3637,.T.);
#19911=EDGE_CURVE('',#15629,#15630,#3638,.T.);
#19912=EDGE_CURVE('',#15630,#15631,#3639,.T.);
#19913=EDGE_CURVE('',#15631,#15632,#3640,.T.);
#19914=EDGE_CURVE('',#15633,#15632,#3641,.T.);
#19915=EDGE_CURVE('',#15633,#15634,#3642,.T.);
#19916=EDGE_CURVE('',#15634,#15635,#3643,.T.);
#19917=EDGE_CURVE('',#15635,#15636,#3644,.T.);
#19918=EDGE_CURVE('',#15637,#15636,#3645,.T.);
#19919=EDGE_CURVE('',#15637,#15638,#3646,.T.);
#19920=EDGE_CURVE('',#15638,#15639,#3647,.T.);
#19921=EDGE_CURVE('',#15639,#15640,#3648,.T.);
#19922=EDGE_CURVE('',#15641,#15640,#3649,.T.);
#19923=EDGE_CURVE('',#15641,#15642,#3650,.T.);
#19924=EDGE_CURVE('',#15642,#15643,#3651,.T.);
#19925=EDGE_CURVE('',#15643,#15644,#3652,.T.);
#19926=EDGE_CURVE('',#15645,#15644,#3653,.T.);
#19927=EDGE_CURVE('',#15645,#15646,#3654,.T.);
#19928=EDGE_CURVE('',#15646,#15647,#3655,.T.);
#19929=EDGE_CURVE('',#15647,#15648,#3656,.T.);
#19930=EDGE_CURVE('',#15649,#15648,#3657,.T.);
#19931=EDGE_CURVE('',#15649,#15650,#3658,.T.);
#19932=EDGE_CURVE('',#15650,#15651,#3659,.T.);
#19933=EDGE_CURVE('',#15651,#15652,#3660,.T.);
#19934=EDGE_CURVE('',#15653,#15652,#3661,.T.);
#19935=EDGE_CURVE('',#15653,#15654,#3662,.T.);
#19936=EDGE_CURVE('',#15654,#15655,#3663,.T.);
#19937=EDGE_CURVE('',#15655,#15656,#3664,.T.);
#19938=EDGE_CURVE('',#15657,#15656,#3665,.T.);
#19939=EDGE_CURVE('',#15657,#15658,#3666,.T.);
#19940=EDGE_CURVE('',#15658,#15659,#3667,.T.);
#19941=EDGE_CURVE('',#15659,#15660,#3668,.T.);
#19942=EDGE_CURVE('',#15661,#15660,#3669,.T.);
#19943=EDGE_CURVE('',#15661,#15662,#3670,.T.);
#19944=EDGE_CURVE('',#15662,#15663,#3671,.T.);
#19945=EDGE_CURVE('',#15663,#15664,#3672,.T.);
#19946=EDGE_CURVE('',#15665,#15664,#3673,.T.);
#19947=EDGE_CURVE('',#15665,#15666,#3674,.T.);
#19948=EDGE_CURVE('',#15666,#15667,#3675,.T.);
#19949=EDGE_CURVE('',#15667,#15668,#3676,.T.);
#19950=EDGE_CURVE('',#15669,#15668,#3677,.T.);
#19951=EDGE_CURVE('',#15669,#15670,#3678,.T.);
#19952=EDGE_CURVE('',#15670,#15671,#3679,.T.);
#19953=EDGE_CURVE('',#15671,#15672,#3680,.T.);
#19954=EDGE_CURVE('',#15673,#15672,#3681,.T.);
#19955=EDGE_CURVE('',#15673,#15674,#3682,.T.);
#19956=EDGE_CURVE('',#15674,#15675,#3683,.T.);
#19957=EDGE_CURVE('',#15675,#15676,#3684,.T.);
#19958=EDGE_CURVE('',#15517,#15676,#3685,.T.);
#19959=EDGE_CURVE('',#15677,#15678,#10033,.T.);
#19960=EDGE_CURVE('',#15514,#15677,#10034,.T.);
#19961=EDGE_CURVE('',#15513,#15678,#10035,.T.);
#19962=EDGE_CURVE('',#15678,#15679,#10036,.T.);
#19963=EDGE_CURVE('',#15679,#15512,#10037,.T.);
#19964=EDGE_CURVE('',#15679,#15680,#3686,.T.);
#19965=EDGE_CURVE('',#15515,#15680,#10038,.T.);
#19966=EDGE_CURVE('',#15680,#15677,#10039,.T.);
#19967=EDGE_CURVE('',#15681,#15518,#10040,.T.);
#19968=EDGE_CURVE('',#15682,#15681,#3687,.T.);
#19969=EDGE_CURVE('',#15682,#15519,#10041,.T.);
#19970=EDGE_CURVE('',#15683,#15682,#3688,.T.);
#19971=EDGE_CURVE('',#15520,#15683,#10042,.T.);
#19972=EDGE_CURVE('',#15684,#15517,#10043,.T.);
#19973=EDGE_CURVE('',#15681,#15684,#3689,.T.);
#19974=EDGE_CURVE('',#15685,#15522,#10044,.T.);
#19975=EDGE_CURVE('',#15686,#15685,#3690,.T.);
#19976=EDGE_CURVE('',#15686,#15523,#10045,.T.);
#19977=EDGE_CURVE('',#15687,#15686,#3691,.T.);
#19978=EDGE_CURVE('',#15524,#15687,#10046,.T.);
#19979=EDGE_CURVE('',#15688,#15521,#10047,.T.);
#19980=EDGE_CURVE('',#15685,#15688,#3692,.T.);
#19981=EDGE_CURVE('',#15689,#15526,#10048,.T.);
#19982=EDGE_CURVE('',#15690,#15689,#3693,.T.);
#19983=EDGE_CURVE('',#15690,#15527,#10049,.T.);
#19984=EDGE_CURVE('',#15691,#15690,#3694,.T.);
#19985=EDGE_CURVE('',#15528,#15691,#10050,.T.);
#19986=EDGE_CURVE('',#15692,#15525,#10051,.T.);
#19987=EDGE_CURVE('',#15689,#15692,#3695,.T.);
#19988=EDGE_CURVE('',#15693,#15530,#10052,.T.);
#19989=EDGE_CURVE('',#15694,#15693,#3696,.T.);
#19990=EDGE_CURVE('',#15694,#15531,#10053,.T.);
#19991=EDGE_CURVE('',#15695,#15694,#3697,.T.);
#19992=EDGE_CURVE('',#15532,#15695,#10054,.T.);
#19993=EDGE_CURVE('',#15696,#15529,#10055,.T.);
#19994=EDGE_CURVE('',#15693,#15696,#3698,.T.);
#19995=EDGE_CURVE('',#15697,#15534,#10056,.T.);
#19996=EDGE_CURVE('',#15698,#15697,#3699,.T.);
#19997=EDGE_CURVE('',#15698,#15535,#10057,.T.);
#19998=EDGE_CURVE('',#15699,#15698,#3700,.T.);
#19999=EDGE_CURVE('',#15536,#15699,#10058,.T.);
#20000=EDGE_CURVE('',#15700,#15533,#10059,.T.);
#20001=EDGE_CURVE('',#15697,#15700,#3701,.T.);
#20002=EDGE_CURVE('',#15701,#15538,#10060,.T.);
#20003=EDGE_CURVE('',#15702,#15701,#3702,.T.);
#20004=EDGE_CURVE('',#15702,#15539,#10061,.T.);
#20005=EDGE_CURVE('',#15703,#15702,#3703,.T.);
#20006=EDGE_CURVE('',#15540,#15703,#10062,.T.);
#20007=EDGE_CURVE('',#15704,#15537,#10063,.T.);
#20008=EDGE_CURVE('',#15701,#15704,#3704,.T.);
#20009=EDGE_CURVE('',#15705,#15542,#10064,.T.);
#20010=EDGE_CURVE('',#15706,#15705,#3705,.T.);
#20011=EDGE_CURVE('',#15706,#15543,#10065,.T.);
#20012=EDGE_CURVE('',#15707,#15706,#3706,.T.);
#20013=EDGE_CURVE('',#15544,#15707,#10066,.T.);
#20014=EDGE_CURVE('',#15708,#15541,#10067,.T.);
#20015=EDGE_CURVE('',#15705,#15708,#3707,.T.);
#20016=EDGE_CURVE('',#15709,#15546,#10068,.T.);
#20017=EDGE_CURVE('',#15710,#15709,#3708,.T.);
#20018=EDGE_CURVE('',#15710,#15547,#10069,.T.);
#20019=EDGE_CURVE('',#15711,#15710,#3709,.T.);
#20020=EDGE_CURVE('',#15548,#15711,#10070,.T.);
#20021=EDGE_CURVE('',#15712,#15545,#10071,.T.);
#20022=EDGE_CURVE('',#15709,#15712,#3710,.T.);
#20023=EDGE_CURVE('',#15713,#15550,#10072,.T.);
#20024=EDGE_CURVE('',#15714,#15713,#3711,.T.);
#20025=EDGE_CURVE('',#15714,#15551,#10073,.T.);
#20026=EDGE_CURVE('',#15715,#15714,#3712,.T.);
#20027=EDGE_CURVE('',#15552,#15715,#10074,.T.);
#20028=EDGE_CURVE('',#15716,#15549,#10075,.T.);
#20029=EDGE_CURVE('',#15713,#15716,#3713,.T.);
#20030=EDGE_CURVE('',#15717,#15554,#10076,.T.);
#20031=EDGE_CURVE('',#15718,#15717,#3714,.T.);
#20032=EDGE_CURVE('',#15718,#15555,#10077,.T.);
#20033=EDGE_CURVE('',#15719,#15718,#3715,.T.);
#20034=EDGE_CURVE('',#15556,#15719,#10078,.T.);
#20035=EDGE_CURVE('',#15720,#15553,#10079,.T.);
#20036=EDGE_CURVE('',#15717,#15720,#3716,.T.);
#20037=EDGE_CURVE('',#15721,#15558,#10080,.T.);
#20038=EDGE_CURVE('',#15722,#15721,#3717,.T.);
#20039=EDGE_CURVE('',#15722,#15559,#10081,.T.);
#20040=EDGE_CURVE('',#15723,#15722,#3718,.T.);
#20041=EDGE_CURVE('',#15560,#15723,#10082,.T.);
#20042=EDGE_CURVE('',#15724,#15557,#10083,.T.);
#20043=EDGE_CURVE('',#15721,#15724,#3719,.T.);
#20044=EDGE_CURVE('',#15725,#15562,#10084,.T.);
#20045=EDGE_CURVE('',#15726,#15725,#3720,.T.);
#20046=EDGE_CURVE('',#15726,#15563,#10085,.T.);
#20047=EDGE_CURVE('',#15727,#15726,#3721,.T.);
#20048=EDGE_CURVE('',#15564,#15727,#10086,.T.);
#20049=EDGE_CURVE('',#15728,#15561,#10087,.T.);
#20050=EDGE_CURVE('',#15725,#15728,#3722,.T.);
#20051=EDGE_CURVE('',#15729,#15566,#10088,.T.);
#20052=EDGE_CURVE('',#15730,#15729,#3723,.T.);
#20053=EDGE_CURVE('',#15730,#15567,#10089,.T.);
#20054=EDGE_CURVE('',#15731,#15730,#3724,.T.);
#20055=EDGE_CURVE('',#15568,#15731,#10090,.T.);
#20056=EDGE_CURVE('',#15732,#15565,#10091,.T.);
#20057=EDGE_CURVE('',#15729,#15732,#3725,.T.);
#20058=EDGE_CURVE('',#15733,#15570,#10092,.T.);
#20059=EDGE_CURVE('',#15734,#15733,#3726,.T.);
#20060=EDGE_CURVE('',#15734,#15571,#10093,.T.);
#20061=EDGE_CURVE('',#15735,#15734,#3727,.T.);
#20062=EDGE_CURVE('',#15572,#15735,#10094,.T.);
#20063=EDGE_CURVE('',#15736,#15569,#10095,.T.);
#20064=EDGE_CURVE('',#15733,#15736,#3728,.T.);
#20065=EDGE_CURVE('',#15737,#15574,#10096,.T.);
#20066=EDGE_CURVE('',#15738,#15737,#3729,.T.);
#20067=EDGE_CURVE('',#15738,#15575,#10097,.T.);
#20068=EDGE_CURVE('',#15739,#15738,#3730,.T.);
#20069=EDGE_CURVE('',#15576,#15739,#10098,.T.);
#20070=EDGE_CURVE('',#15740,#15573,#10099,.T.);
#20071=EDGE_CURVE('',#15737,#15740,#3731,.T.);
#20072=EDGE_CURVE('',#15741,#15578,#10100,.T.);
#20073=EDGE_CURVE('',#15742,#15741,#3732,.T.);
#20074=EDGE_CURVE('',#15742,#15579,#10101,.T.);
#20075=EDGE_CURVE('',#15743,#15742,#3733,.T.);
#20076=EDGE_CURVE('',#15580,#15743,#10102,.T.);
#20077=EDGE_CURVE('',#15744,#15577,#10103,.T.);
#20078=EDGE_CURVE('',#15741,#15744,#3734,.T.);
#20079=EDGE_CURVE('',#15745,#15582,#10104,.T.);
#20080=EDGE_CURVE('',#15746,#15745,#3735,.T.);
#20081=EDGE_CURVE('',#15746,#15583,#10105,.T.);
#20082=EDGE_CURVE('',#15747,#15746,#3736,.T.);
#20083=EDGE_CURVE('',#15584,#15747,#10106,.T.);
#20084=EDGE_CURVE('',#15748,#15581,#10107,.T.);
#20085=EDGE_CURVE('',#15745,#15748,#3737,.T.);
#20086=EDGE_CURVE('',#15749,#15586,#10108,.T.);
#20087=EDGE_CURVE('',#15750,#15749,#3738,.T.);
#20088=EDGE_CURVE('',#15750,#15587,#10109,.T.);
#20089=EDGE_CURVE('',#15751,#15750,#3739,.T.);
#20090=EDGE_CURVE('',#15588,#15751,#10110,.T.);
#20091=EDGE_CURVE('',#15752,#15585,#10111,.T.);
#20092=EDGE_CURVE('',#15749,#15752,#3740,.T.);
#20093=EDGE_CURVE('',#15753,#15590,#10112,.T.);
#20094=EDGE_CURVE('',#15754,#15753,#3741,.T.);
#20095=EDGE_CURVE('',#15754,#15591,#10113,.T.);
#20096=EDGE_CURVE('',#15755,#15754,#3742,.T.);
#20097=EDGE_CURVE('',#15592,#15755,#10114,.T.);
#20098=EDGE_CURVE('',#15756,#15589,#10115,.T.);
#20099=EDGE_CURVE('',#15753,#15756,#3743,.T.);
#20100=EDGE_CURVE('',#15757,#15594,#10116,.T.);
#20101=EDGE_CURVE('',#15758,#15757,#3744,.T.);
#20102=EDGE_CURVE('',#15758,#15595,#10117,.T.);
#20103=EDGE_CURVE('',#15759,#15758,#3745,.T.);
#20104=EDGE_CURVE('',#15596,#15759,#10118,.T.);
#20105=EDGE_CURVE('',#15760,#15593,#10119,.T.);
#20106=EDGE_CURVE('',#15757,#15760,#3746,.T.);
#20107=EDGE_CURVE('',#15761,#15598,#10120,.T.);
#20108=EDGE_CURVE('',#15762,#15761,#3747,.T.);
#20109=EDGE_CURVE('',#15762,#15599,#10121,.T.);
#20110=EDGE_CURVE('',#15763,#15762,#3748,.T.);
#20111=EDGE_CURVE('',#15600,#15763,#10122,.T.);
#20112=EDGE_CURVE('',#15764,#15597,#10123,.T.);
#20113=EDGE_CURVE('',#15761,#15764,#3749,.T.);
#20114=EDGE_CURVE('',#15765,#15602,#10124,.T.);
#20115=EDGE_CURVE('',#15766,#15765,#3750,.T.);
#20116=EDGE_CURVE('',#15766,#15603,#10125,.T.);
#20117=EDGE_CURVE('',#15767,#15766,#3751,.T.);
#20118=EDGE_CURVE('',#15604,#15767,#10126,.T.);
#20119=EDGE_CURVE('',#15768,#15601,#10127,.T.);
#20120=EDGE_CURVE('',#15765,#15768,#3752,.T.);
#20121=EDGE_CURVE('',#15769,#15606,#10128,.T.);
#20122=EDGE_CURVE('',#15770,#15769,#3753,.T.);
#20123=EDGE_CURVE('',#15770,#15607,#10129,.T.);
#20124=EDGE_CURVE('',#15771,#15770,#3754,.T.);
#20125=EDGE_CURVE('',#15608,#15771,#10130,.T.);
#20126=EDGE_CURVE('',#15772,#15605,#10131,.T.);
#20127=EDGE_CURVE('',#15769,#15772,#3755,.T.);
#20128=EDGE_CURVE('',#15773,#15610,#10132,.T.);
#20129=EDGE_CURVE('',#15774,#15773,#3756,.T.);
#20130=EDGE_CURVE('',#15774,#15611,#10133,.T.);
#20131=EDGE_CURVE('',#15775,#15774,#3757,.T.);
#20132=EDGE_CURVE('',#15612,#15775,#10134,.T.);
#20133=EDGE_CURVE('',#15776,#15609,#10135,.T.);
#20134=EDGE_CURVE('',#15773,#15776,#3758,.T.);
#20135=EDGE_CURVE('',#15777,#15614,#10136,.T.);
#20136=EDGE_CURVE('',#15778,#15777,#3759,.T.);
#20137=EDGE_CURVE('',#15778,#15615,#10137,.T.);
#20138=EDGE_CURVE('',#15779,#15778,#3760,.T.);
#20139=EDGE_CURVE('',#15616,#15779,#10138,.T.);
#20140=EDGE_CURVE('',#15780,#15613,#10139,.T.);
#20141=EDGE_CURVE('',#15777,#15780,#3761,.T.);
#20142=EDGE_CURVE('',#15781,#15618,#10140,.T.);
#20143=EDGE_CURVE('',#15782,#15781,#3762,.T.);
#20144=EDGE_CURVE('',#15782,#15619,#10141,.T.);
#20145=EDGE_CURVE('',#15783,#15782,#3763,.T.);
#20146=EDGE_CURVE('',#15620,#15783,#10142,.T.);
#20147=EDGE_CURVE('',#15784,#15617,#10143,.T.);
#20148=EDGE_CURVE('',#15781,#15784,#3764,.T.);
#20149=EDGE_CURVE('',#15785,#15622,#10144,.T.);
#20150=EDGE_CURVE('',#15786,#15785,#3765,.T.);
#20151=EDGE_CURVE('',#15786,#15623,#10145,.T.);
#20152=EDGE_CURVE('',#15787,#15786,#3766,.T.);
#20153=EDGE_CURVE('',#15624,#15787,#10146,.T.);
#20154=EDGE_CURVE('',#15788,#15621,#10147,.T.);
#20155=EDGE_CURVE('',#15785,#15788,#3767,.T.);
#20156=EDGE_CURVE('',#15789,#15626,#10148,.T.);
#20157=EDGE_CURVE('',#15790,#15789,#3768,.T.);
#20158=EDGE_CURVE('',#15790,#15627,#10149,.T.);
#20159=EDGE_CURVE('',#15791,#15790,#3769,.T.);
#20160=EDGE_CURVE('',#15628,#15791,#10150,.T.);
#20161=EDGE_CURVE('',#15792,#15625,#10151,.T.);
#20162=EDGE_CURVE('',#15789,#15792,#3770,.T.);
#20163=EDGE_CURVE('',#15793,#15630,#10152,.T.);
#20164=EDGE_CURVE('',#15794,#15793,#3771,.T.);
#20165=EDGE_CURVE('',#15794,#15631,#10153,.T.);
#20166=EDGE_CURVE('',#15795,#15794,#3772,.T.);
#20167=EDGE_CURVE('',#15632,#15795,#10154,.T.);
#20168=EDGE_CURVE('',#15796,#15629,#10155,.T.);
#20169=EDGE_CURVE('',#15793,#15796,#3773,.T.);
#20170=EDGE_CURVE('',#15797,#15634,#10156,.T.);
#20171=EDGE_CURVE('',#15798,#15797,#3774,.T.);
#20172=EDGE_CURVE('',#15798,#15635,#10157,.T.);
#20173=EDGE_CURVE('',#15799,#15798,#3775,.T.);
#20174=EDGE_CURVE('',#15636,#15799,#10158,.T.);
#20175=EDGE_CURVE('',#15800,#15633,#10159,.T.);
#20176=EDGE_CURVE('',#15797,#15800,#3776,.T.);
#20177=EDGE_CURVE('',#15801,#15638,#10160,.T.);
#20178=EDGE_CURVE('',#15802,#15801,#3777,.T.);
#20179=EDGE_CURVE('',#15802,#15639,#10161,.T.);
#20180=EDGE_CURVE('',#15803,#15802,#3778,.T.);
#20181=EDGE_CURVE('',#15640,#15803,#10162,.T.);
#20182=EDGE_CURVE('',#15804,#15637,#10163,.T.);
#20183=EDGE_CURVE('',#15801,#15804,#3779,.T.);
#20184=EDGE_CURVE('',#15805,#15642,#10164,.T.);
#20185=EDGE_CURVE('',#15806,#15805,#3780,.T.);
#20186=EDGE_CURVE('',#15806,#15643,#10165,.T.);
#20187=EDGE_CURVE('',#15807,#15806,#3781,.T.);
#20188=EDGE_CURVE('',#15644,#15807,#10166,.T.);
#20189=EDGE_CURVE('',#15808,#15641,#10167,.T.);
#20190=EDGE_CURVE('',#15805,#15808,#3782,.T.);
#20191=EDGE_CURVE('',#15809,#15646,#10168,.T.);
#20192=EDGE_CURVE('',#15810,#15809,#3783,.T.);
#20193=EDGE_CURVE('',#15810,#15647,#10169,.T.);
#20194=EDGE_CURVE('',#15811,#15810,#3784,.T.);
#20195=EDGE_CURVE('',#15648,#15811,#10170,.T.);
#20196=EDGE_CURVE('',#15812,#15645,#10171,.T.);
#20197=EDGE_CURVE('',#15809,#15812,#3785,.T.);
#20198=EDGE_CURVE('',#15813,#15650,#10172,.T.);
#20199=EDGE_CURVE('',#15814,#15813,#3786,.T.);
#20200=EDGE_CURVE('',#15814,#15651,#10173,.T.);
#20201=EDGE_CURVE('',#15815,#15814,#3787,.T.);
#20202=EDGE_CURVE('',#15652,#15815,#10174,.T.);
#20203=EDGE_CURVE('',#15816,#15649,#10175,.T.);
#20204=EDGE_CURVE('',#15813,#15816,#3788,.T.);
#20205=EDGE_CURVE('',#15817,#15654,#10176,.T.);
#20206=EDGE_CURVE('',#15818,#15817,#3789,.T.);
#20207=EDGE_CURVE('',#15818,#15655,#10177,.T.);
#20208=EDGE_CURVE('',#15819,#15818,#3790,.T.);
#20209=EDGE_CURVE('',#15656,#15819,#10178,.T.);
#20210=EDGE_CURVE('',#15820,#15653,#10179,.T.);
#20211=EDGE_CURVE('',#15817,#15820,#3791,.T.);
#20212=EDGE_CURVE('',#15821,#15658,#10180,.T.);
#20213=EDGE_CURVE('',#15822,#15821,#3792,.T.);
#20214=EDGE_CURVE('',#15822,#15659,#10181,.T.);
#20215=EDGE_CURVE('',#15823,#15822,#3793,.T.);
#20216=EDGE_CURVE('',#15660,#15823,#10182,.T.);
#20217=EDGE_CURVE('',#15824,#15657,#10183,.T.);
#20218=EDGE_CURVE('',#15821,#15824,#3794,.T.);
#20219=EDGE_CURVE('',#15825,#15662,#10184,.T.);
#20220=EDGE_CURVE('',#15826,#15825,#3795,.T.);
#20221=EDGE_CURVE('',#15826,#15663,#10185,.T.);
#20222=EDGE_CURVE('',#15827,#15826,#3796,.T.);
#20223=EDGE_CURVE('',#15664,#15827,#10186,.T.);
#20224=EDGE_CURVE('',#15828,#15661,#10187,.T.);
#20225=EDGE_CURVE('',#15825,#15828,#3797,.T.);
#20226=EDGE_CURVE('',#15829,#15666,#10188,.T.);
#20227=EDGE_CURVE('',#15830,#15829,#3798,.T.);
#20228=EDGE_CURVE('',#15830,#15667,#10189,.T.);
#20229=EDGE_CURVE('',#15831,#15830,#3799,.T.);
#20230=EDGE_CURVE('',#15668,#15831,#10190,.T.);
#20231=EDGE_CURVE('',#15832,#15665,#10191,.T.);
#20232=EDGE_CURVE('',#15829,#15832,#3800,.T.);
#20233=EDGE_CURVE('',#15833,#15670,#10192,.T.);
#20234=EDGE_CURVE('',#15834,#15833,#3801,.T.);
#20235=EDGE_CURVE('',#15834,#15671,#10193,.T.);
#20236=EDGE_CURVE('',#15835,#15834,#3802,.T.);
#20237=EDGE_CURVE('',#15672,#15835,#10194,.T.);
#20238=EDGE_CURVE('',#15836,#15669,#10195,.T.);
#20239=EDGE_CURVE('',#15833,#15836,#3803,.T.);
#20240=EDGE_CURVE('',#15837,#15835,#3804,.T.);
#20241=EDGE_CURVE('',#15837,#15673,#10196,.T.);
#20242=EDGE_CURVE('',#15836,#15831,#3805,.T.);
#20243=EDGE_CURVE('',#15832,#15827,#3806,.T.);
#20244=EDGE_CURVE('',#15828,#15823,#3807,.T.);
#20245=EDGE_CURVE('',#15824,#15819,#3808,.T.);
#20246=EDGE_CURVE('',#15820,#15815,#3809,.T.);
#20247=EDGE_CURVE('',#15816,#15811,#3810,.T.);
#20248=EDGE_CURVE('',#15812,#15807,#3811,.T.);
#20249=EDGE_CURVE('',#15808,#15803,#3812,.T.);
#20250=EDGE_CURVE('',#15804,#15799,#3813,.T.);
#20251=EDGE_CURVE('',#15800,#15795,#3814,.T.);
#20252=EDGE_CURVE('',#15796,#15791,#3815,.T.);
#20253=EDGE_CURVE('',#15792,#15787,#3816,.T.);
#20254=EDGE_CURVE('',#15788,#15783,#3817,.T.);
#20255=EDGE_CURVE('',#15784,#15779,#3818,.T.);
#20256=EDGE_CURVE('',#15780,#15775,#3819,.T.);
#20257=EDGE_CURVE('',#15776,#15771,#3820,.T.);
#20258=EDGE_CURVE('',#15772,#15767,#3821,.T.);
#20259=EDGE_CURVE('',#15768,#15763,#3822,.T.);
#20260=EDGE_CURVE('',#15764,#15759,#3823,.T.);
#20261=EDGE_CURVE('',#15760,#15755,#3824,.T.);
#20262=EDGE_CURVE('',#15756,#15751,#3825,.T.);
#20263=EDGE_CURVE('',#15752,#15747,#3826,.T.);
#20264=EDGE_CURVE('',#15748,#15743,#3827,.T.);
#20265=EDGE_CURVE('',#15744,#15739,#3828,.T.);
#20266=EDGE_CURVE('',#15740,#15735,#3829,.T.);
#20267=EDGE_CURVE('',#15736,#15731,#3830,.T.);
#20268=EDGE_CURVE('',#15732,#15727,#3831,.T.);
#20269=EDGE_CURVE('',#15728,#15723,#3832,.T.);
#20270=EDGE_CURVE('',#15724,#15719,#3833,.T.);
#20271=EDGE_CURVE('',#15720,#15715,#3834,.T.);
#20272=EDGE_CURVE('',#15716,#15711,#3835,.T.);
#20273=EDGE_CURVE('',#15712,#15707,#3836,.T.);
#20274=EDGE_CURVE('',#15708,#15703,#3837,.T.);
#20275=EDGE_CURVE('',#15704,#15699,#3838,.T.);
#20276=EDGE_CURVE('',#15700,#15695,#3839,.T.);
#20277=EDGE_CURVE('',#15696,#15691,#3840,.T.);
#20278=EDGE_CURVE('',#15692,#15687,#3841,.T.);
#20279=EDGE_CURVE('',#15688,#15683,#3842,.T.);
#20280=EDGE_CURVE('',#15838,#15674,#10197,.T.);
#20281=EDGE_CURVE('',#15839,#15838,#3843,.T.);
#20282=EDGE_CURVE('',#15839,#15675,#10198,.T.);
#20283=EDGE_CURVE('',#15840,#15839,#3844,.T.);
#20284=EDGE_CURVE('',#15676,#15840,#10199,.T.);
#20285=EDGE_CURVE('',#15838,#15837,#3845,.T.);
#20286=EDGE_CURVE('',#15684,#15840,#3846,.T.);
#27770=ORIENTED_EDGE('',*,*,#19787,.T.);
#27771=ORIENTED_EDGE('',*,*,#19788,.T.);
#27772=ORIENTED_EDGE('',*,*,#19789,.T.);
#27773=ORIENTED_EDGE('',*,*,#19790,.T.);
#27774=ORIENTED_EDGE('',*,*,#19788,.F.);
#27775=ORIENTED_EDGE('',*,*,#19790,.F.);
#27776=ORIENTED_EDGE('',*,*,#19791,.T.);
#27777=ORIENTED_EDGE('',*,*,#19792,.F.);
#27778=ORIENTED_EDGE('',*,*,#19791,.F.);
#27779=ORIENTED_EDGE('',*,*,#19789,.F.);
#27780=ORIENTED_EDGE('',*,*,#19787,.F.);
#27781=ORIENTED_EDGE('',*,*,#19793,.T.);
#27782=ORIENTED_EDGE('',*,*,#19794,.T.);
#27783=ORIENTED_EDGE('',*,*,#19795,.T.);
#27784=ORIENTED_EDGE('',*,*,#19796,.T.);
#27785=ORIENTED_EDGE('',*,*,#19797,.T.);
#27786=ORIENTED_EDGE('',*,*,#19798,.T.);
#27787=ORIENTED_EDGE('',*,*,#19792,.T.);
#27788=ORIENTED_EDGE('',*,*,#19798,.F.);
#27789=ORIENTED_EDGE('',*,*,#19799,.T.);
#27790=ORIENTED_EDGE('',*,*,#19800,.T.);
#27791=ORIENTED_EDGE('',*,*,#19801,.T.);
#27792=ORIENTED_EDGE('',*,*,#19802,.F.);
#27793=ORIENTED_EDGE('',*,*,#19803,.T.);
#27794=ORIENTED_EDGE('',*,*,#19804,.T.);
#27795=ORIENTED_EDGE('',*,*,#19805,.T.);
#27796=ORIENTED_EDGE('',*,*,#19806,.F.);
#27797=ORIENTED_EDGE('',*,*,#19807,.T.);
#27798=ORIENTED_EDGE('',*,*,#19808,.T.);
#27799=ORIENTED_EDGE('',*,*,#19809,.T.);
#27800=ORIENTED_EDGE('',*,*,#19810,.F.);
#27801=ORIENTED_EDGE('',*,*,#19811,.T.);
#27802=ORIENTED_EDGE('',*,*,#19812,.T.);
#27803=ORIENTED_EDGE('',*,*,#19813,.T.);
#27804=ORIENTED_EDGE('',*,*,#19814,.F.);
#27805=ORIENTED_EDGE('',*,*,#19815,.T.);
#27806=ORIENTED_EDGE('',*,*,#19816,.T.);
#27807=ORIENTED_EDGE('',*,*,#19817,.T.);
#27808=ORIENTED_EDGE('',*,*,#19818,.F.);
#27809=ORIENTED_EDGE('',*,*,#19819,.T.);
#27810=ORIENTED_EDGE('',*,*,#19820,.T.);
#27811=ORIENTED_EDGE('',*,*,#19821,.T.);
#27812=ORIENTED_EDGE('',*,*,#19822,.F.);
#27813=ORIENTED_EDGE('',*,*,#19823,.T.);
#27814=ORIENTED_EDGE('',*,*,#19824,.T.);
#27815=ORIENTED_EDGE('',*,*,#19825,.T.);
#27816=ORIENTED_EDGE('',*,*,#19826,.F.);
#27817=ORIENTED_EDGE('',*,*,#19827,.T.);
#27818=ORIENTED_EDGE('',*,*,#19828,.T.);
#27819=ORIENTED_EDGE('',*,*,#19829,.T.);
#27820=ORIENTED_EDGE('',*,*,#19830,.F.);
#27821=ORIENTED_EDGE('',*,*,#19831,.T.);
#27822=ORIENTED_EDGE('',*,*,#19832,.T.);
#27823=ORIENTED_EDGE('',*,*,#19833,.T.);
#27824=ORIENTED_EDGE('',*,*,#19834,.F.);
#27825=ORIENTED_EDGE('',*,*,#19835,.T.);
#27826=ORIENTED_EDGE('',*,*,#19836,.T.);
#27827=ORIENTED_EDGE('',*,*,#19837,.T.);
#27828=ORIENTED_EDGE('',*,*,#19838,.F.);
#27829=ORIENTED_EDGE('',*,*,#19839,.T.);
#27830=ORIENTED_EDGE('',*,*,#19840,.T.);
#27831=ORIENTED_EDGE('',*,*,#19841,.T.);
#27832=ORIENTED_EDGE('',*,*,#19842,.F.);
#27833=ORIENTED_EDGE('',*,*,#19843,.T.);
#27834=ORIENTED_EDGE('',*,*,#19844,.T.);
#27835=ORIENTED_EDGE('',*,*,#19845,.T.);
#27836=ORIENTED_EDGE('',*,*,#19846,.F.);
#27837=ORIENTED_EDGE('',*,*,#19847,.T.);
#27838=ORIENTED_EDGE('',*,*,#19848,.T.);
#27839=ORIENTED_EDGE('',*,*,#19849,.T.);
#27840=ORIENTED_EDGE('',*,*,#19850,.F.);
#27841=ORIENTED_EDGE('',*,*,#19851,.T.);
#27842=ORIENTED_EDGE('',*,*,#19852,.T.);
#27843=ORIENTED_EDGE('',*,*,#19853,.T.);
#27844=ORIENTED_EDGE('',*,*,#19854,.F.);
#27845=ORIENTED_EDGE('',*,*,#19855,.T.);
#27846=ORIENTED_EDGE('',*,*,#19856,.T.);
#27847=ORIENTED_EDGE('',*,*,#19857,.T.);
#27848=ORIENTED_EDGE('',*,*,#19858,.F.);
#27849=ORIENTED_EDGE('',*,*,#19859,.T.);
#27850=ORIENTED_EDGE('',*,*,#19860,.T.);
#27851=ORIENTED_EDGE('',*,*,#19861,.T.);
#27852=ORIENTED_EDGE('',*,*,#19862,.F.);
#27853=ORIENTED_EDGE('',*,*,#19863,.T.);
#27854=ORIENTED_EDGE('',*,*,#19864,.T.);
#27855=ORIENTED_EDGE('',*,*,#19865,.T.);
#27856=ORIENTED_EDGE('',*,*,#19866,.F.);
#27857=ORIENTED_EDGE('',*,*,#19867,.T.);
#27858=ORIENTED_EDGE('',*,*,#19868,.T.);
#27859=ORIENTED_EDGE('',*,*,#19869,.T.);
#27860=ORIENTED_EDGE('',*,*,#19870,.F.);
#27861=ORIENTED_EDGE('',*,*,#19871,.T.);
#27862=ORIENTED_EDGE('',*,*,#19872,.T.);
#27863=ORIENTED_EDGE('',*,*,#19873,.T.);
#27864=ORIENTED_EDGE('',*,*,#19874,.F.);
#27865=ORIENTED_EDGE('',*,*,#19875,.T.);
#27866=ORIENTED_EDGE('',*,*,#19876,.T.);
#27867=ORIENTED_EDGE('',*,*,#19877,.T.);
#27868=ORIENTED_EDGE('',*,*,#19878,.F.);
#27869=ORIENTED_EDGE('',*,*,#19879,.T.);
#27870=ORIENTED_EDGE('',*,*,#19880,.T.);
#27871=ORIENTED_EDGE('',*,*,#19881,.T.);
#27872=ORIENTED_EDGE('',*,*,#19882,.F.);
#27873=ORIENTED_EDGE('',*,*,#19883,.T.);
#27874=ORIENTED_EDGE('',*,*,#19884,.T.);
#27875=ORIENTED_EDGE('',*,*,#19885,.T.);
#27876=ORIENTED_EDGE('',*,*,#19886,.F.);
#27877=ORIENTED_EDGE('',*,*,#19887,.T.);
#27878=ORIENTED_EDGE('',*,*,#19888,.T.);
#27879=ORIENTED_EDGE('',*,*,#19889,.T.);
#27880=ORIENTED_EDGE('',*,*,#19890,.F.);
#27881=ORIENTED_EDGE('',*,*,#19891,.T.);
#27882=ORIENTED_EDGE('',*,*,#19892,.T.);
#27883=ORIENTED_EDGE('',*,*,#19893,.T.);
#27884=ORIENTED_EDGE('',*,*,#19894,.F.);
#27885=ORIENTED_EDGE('',*,*,#19895,.T.);
#27886=ORIENTED_EDGE('',*,*,#19896,.T.);
#27887=ORIENTED_EDGE('',*,*,#19897,.T.);
#27888=ORIENTED_EDGE('',*,*,#19898,.F.);
#27889=ORIENTED_EDGE('',*,*,#19899,.T.);
#27890=ORIENTED_EDGE('',*,*,#19900,.T.);
#27891=ORIENTED_EDGE('',*,*,#19901,.T.);
#27892=ORIENTED_EDGE('',*,*,#19902,.F.);
#27893=ORIENTED_EDGE('',*,*,#19903,.T.);
#27894=ORIENTED_EDGE('',*,*,#19904,.T.);
#27895=ORIENTED_EDGE('',*,*,#19905,.T.);
#27896=ORIENTED_EDGE('',*,*,#19906,.F.);
#27897=ORIENTED_EDGE('',*,*,#19907,.T.);
#27898=ORIENTED_EDGE('',*,*,#19908,.T.);
#27899=ORIENTED_EDGE('',*,*,#19909,.T.);
#27900=ORIENTED_EDGE('',*,*,#19910,.F.);
#27901=ORIENTED_EDGE('',*,*,#19911,.T.);
#27902=ORIENTED_EDGE('',*,*,#19912,.T.);
#27903=ORIENTED_EDGE('',*,*,#19913,.T.);
#27904=ORIENTED_EDGE('',*,*,#19914,.F.);
#27905=ORIENTED_EDGE('',*,*,#19915,.T.);
#27906=ORIENTED_EDGE('',*,*,#19916,.T.);
#27907=ORIENTED_EDGE('',*,*,#19917,.T.);
#27908=ORIENTED_EDGE('',*,*,#19918,.F.);
#27909=ORIENTED_EDGE('',*,*,#19919,.T.);
#27910=ORIENTED_EDGE('',*,*,#19920,.T.);
#27911=ORIENTED_EDGE('',*,*,#19921,.T.);
#27912=ORIENTED_EDGE('',*,*,#19922,.F.);
#27913=ORIENTED_EDGE('',*,*,#19923,.T.);
#27914=ORIENTED_EDGE('',*,*,#19924,.T.);
#27915=ORIENTED_EDGE('',*,*,#19925,.T.);
#27916=ORIENTED_EDGE('',*,*,#19926,.F.);
#27917=ORIENTED_EDGE('',*,*,#19927,.T.);
#27918=ORIENTED_EDGE('',*,*,#19928,.T.);
#27919=ORIENTED_EDGE('',*,*,#19929,.T.);
#27920=ORIENTED_EDGE('',*,*,#19930,.F.);
#27921=ORIENTED_EDGE('',*,*,#19931,.T.);
#27922=ORIENTED_EDGE('',*,*,#19932,.T.);
#27923=ORIENTED_EDGE('',*,*,#19933,.T.);
#27924=ORIENTED_EDGE('',*,*,#19934,.F.);
#27925=ORIENTED_EDGE('',*,*,#19935,.T.);
#27926=ORIENTED_EDGE('',*,*,#19936,.T.);
#27927=ORIENTED_EDGE('',*,*,#19937,.T.);
#27928=ORIENTED_EDGE('',*,*,#19938,.F.);
#27929=ORIENTED_EDGE('',*,*,#19939,.T.);
#27930=ORIENTED_EDGE('',*,*,#19940,.T.);
#27931=ORIENTED_EDGE('',*,*,#19941,.T.);
#27932=ORIENTED_EDGE('',*,*,#19942,.F.);
#27933=ORIENTED_EDGE('',*,*,#19943,.T.);
#27934=ORIENTED_EDGE('',*,*,#19944,.T.);
#27935=ORIENTED_EDGE('',*,*,#19945,.T.);
#27936=ORIENTED_EDGE('',*,*,#19946,.F.);
#27937=ORIENTED_EDGE('',*,*,#19947,.T.);
#27938=ORIENTED_EDGE('',*,*,#19948,.T.);
#27939=ORIENTED_EDGE('',*,*,#19949,.T.);
#27940=ORIENTED_EDGE('',*,*,#19950,.F.);
#27941=ORIENTED_EDGE('',*,*,#19951,.T.);
#27942=ORIENTED_EDGE('',*,*,#19952,.T.);
#27943=ORIENTED_EDGE('',*,*,#19953,.T.);
#27944=ORIENTED_EDGE('',*,*,#19954,.F.);
#27945=ORIENTED_EDGE('',*,*,#19955,.T.);
#27946=ORIENTED_EDGE('',*,*,#19956,.T.);
#27947=ORIENTED_EDGE('',*,*,#19957,.T.);
#27948=ORIENTED_EDGE('',*,*,#19958,.F.);
#27949=ORIENTED_EDGE('',*,*,#19797,.F.);
#27950=ORIENTED_EDGE('',*,*,#19959,.F.);
#27951=ORIENTED_EDGE('',*,*,#19960,.F.);
#27952=ORIENTED_EDGE('',*,*,#19794,.F.);
#27953=ORIENTED_EDGE('',*,*,#19961,.T.);
#27954=ORIENTED_EDGE('',*,*,#19962,.F.);
#27955=ORIENTED_EDGE('',*,*,#19961,.F.);
#27956=ORIENTED_EDGE('',*,*,#19793,.F.);
#27957=ORIENTED_EDGE('',*,*,#19963,.F.);
#27958=ORIENTED_EDGE('',*,*,#19964,.F.);
#27959=ORIENTED_EDGE('',*,*,#19963,.T.);
#27960=ORIENTED_EDGE('',*,*,#19796,.F.);
#27961=ORIENTED_EDGE('',*,*,#19965,.T.);
#27962=ORIENTED_EDGE('',*,*,#19966,.F.);
#27963=ORIENTED_EDGE('',*,*,#19965,.F.);
#27964=ORIENTED_EDGE('',*,*,#19795,.F.);
#27965=ORIENTED_EDGE('',*,*,#19960,.T.);
#27966=ORIENTED_EDGE('',*,*,#19800,.F.);
#27967=ORIENTED_EDGE('',*,*,#19967,.F.);
#27968=ORIENTED_EDGE('',*,*,#19968,.F.);
#27969=ORIENTED_EDGE('',*,*,#19969,.T.);
#27970=ORIENTED_EDGE('',*,*,#19801,.F.);
#27971=ORIENTED_EDGE('',*,*,#19969,.F.);
#27972=ORIENTED_EDGE('',*,*,#19970,.F.);
#27973=ORIENTED_EDGE('',*,*,#19971,.F.);
#27974=ORIENTED_EDGE('',*,*,#19799,.F.);
#27975=ORIENTED_EDGE('',*,*,#19972,.F.);
#27976=ORIENTED_EDGE('',*,*,#19973,.F.);
#27977=ORIENTED_EDGE('',*,*,#19967,.T.);
#27978=ORIENTED_EDGE('',*,*,#19804,.F.);
#27979=ORIENTED_EDGE('',*,*,#19974,.F.);
#27980=ORIENTED_EDGE('',*,*,#19975,.F.);
#27981=ORIENTED_EDGE('',*,*,#19976,.T.);
#27982=ORIENTED_EDGE('',*,*,#19805,.F.);
#27983=ORIENTED_EDGE('',*,*,#19976,.F.);
#27984=ORIENTED_EDGE('',*,*,#19977,.F.);
#27985=ORIENTED_EDGE('',*,*,#19978,.F.);
#27986=ORIENTED_EDGE('',*,*,#19803,.F.);
#27987=ORIENTED_EDGE('',*,*,#19979,.F.);
#27988=ORIENTED_EDGE('',*,*,#19980,.F.);
#27989=ORIENTED_EDGE('',*,*,#19974,.T.);
#27990=ORIENTED_EDGE('',*,*,#19808,.F.);
#27991=ORIENTED_EDGE('',*,*,#19981,.F.);
#27992=ORIENTED_EDGE('',*,*,#19982,.F.);
#27993=ORIENTED_EDGE('',*,*,#19983,.T.);
#27994=ORIENTED_EDGE('',*,*,#19809,.F.);
#27995=ORIENTED_EDGE('',*,*,#19983,.F.);
#27996=ORIENTED_EDGE('',*,*,#19984,.F.);
#27997=ORIENTED_EDGE('',*,*,#19985,.F.);
#27998=ORIENTED_EDGE('',*,*,#19807,.F.);
#27999=ORIENTED_EDGE('',*,*,#19986,.F.);
#28000=ORIENTED_EDGE('',*,*,#19987,.F.);
#28001=ORIENTED_EDGE('',*,*,#19981,.T.);
#28002=ORIENTED_EDGE('',*,*,#19812,.F.);
#28003=ORIENTED_EDGE('',*,*,#19988,.F.);
#28004=ORIENTED_EDGE('',*,*,#19989,.F.);
#28005=ORIENTED_EDGE('',*,*,#19990,.T.);
#28006=ORIENTED_EDGE('',*,*,#19813,.F.);
#28007=ORIENTED_EDGE('',*,*,#19990,.F.);
#28008=ORIENTED_EDGE('',*,*,#19991,.F.);
#28009=ORIENTED_EDGE('',*,*,#19992,.F.);
#28010=ORIENTED_EDGE('',*,*,#19811,.F.);
#28011=ORIENTED_EDGE('',*,*,#19993,.F.);
#28012=ORIENTED_EDGE('',*,*,#19994,.F.);
#28013=ORIENTED_EDGE('',*,*,#19988,.T.);
#28014=ORIENTED_EDGE('',*,*,#19816,.F.);
#28015=ORIENTED_EDGE('',*,*,#19995,.F.);
#28016=ORIENTED_EDGE('',*,*,#19996,.F.);
#28017=ORIENTED_EDGE('',*,*,#19997,.T.);
#28018=ORIENTED_EDGE('',*,*,#19817,.F.);
#28019=ORIENTED_EDGE('',*,*,#19997,.F.);
#28020=ORIENTED_EDGE('',*,*,#19998,.F.);
#28021=ORIENTED_EDGE('',*,*,#19999,.F.);
#28022=ORIENTED_EDGE('',*,*,#19815,.F.);
#28023=ORIENTED_EDGE('',*,*,#20000,.F.);
#28024=ORIENTED_EDGE('',*,*,#20001,.F.);
#28025=ORIENTED_EDGE('',*,*,#19995,.T.);
#28026=ORIENTED_EDGE('',*,*,#19820,.F.);
#28027=ORIENTED_EDGE('',*,*,#20002,.F.);
#28028=ORIENTED_EDGE('',*,*,#20003,.F.);
#28029=ORIENTED_EDGE('',*,*,#20004,.T.);
#28030=ORIENTED_EDGE('',*,*,#19821,.F.);
#28031=ORIENTED_EDGE('',*,*,#20004,.F.);
#28032=ORIENTED_EDGE('',*,*,#20005,.F.);
#28033=ORIENTED_EDGE('',*,*,#20006,.F.);
#28034=ORIENTED_EDGE('',*,*,#19819,.F.);
#28035=ORIENTED_EDGE('',*,*,#20007,.F.);
#28036=ORIENTED_EDGE('',*,*,#20008,.F.);
#28037=ORIENTED_EDGE('',*,*,#20002,.T.);
#28038=ORIENTED_EDGE('',*,*,#19824,.F.);
#28039=ORIENTED_EDGE('',*,*,#20009,.F.);
#28040=ORIENTED_EDGE('',*,*,#20010,.F.);
#28041=ORIENTED_EDGE('',*,*,#20011,.T.);
#28042=ORIENTED_EDGE('',*,*,#19825,.F.);
#28043=ORIENTED_EDGE('',*,*,#20011,.F.);
#28044=ORIENTED_EDGE('',*,*,#20012,.F.);
#28045=ORIENTED_EDGE('',*,*,#20013,.F.);
#28046=ORIENTED_EDGE('',*,*,#19823,.F.);
#28047=ORIENTED_EDGE('',*,*,#20014,.F.);
#28048=ORIENTED_EDGE('',*,*,#20015,.F.);
#28049=ORIENTED_EDGE('',*,*,#20009,.T.);
#28050=ORIENTED_EDGE('',*,*,#19828,.F.);
#28051=ORIENTED_EDGE('',*,*,#20016,.F.);
#28052=ORIENTED_EDGE('',*,*,#20017,.F.);
#28053=ORIENTED_EDGE('',*,*,#20018,.T.);
#28054=ORIENTED_EDGE('',*,*,#19829,.F.);
#28055=ORIENTED_EDGE('',*,*,#20018,.F.);
#28056=ORIENTED_EDGE('',*,*,#20019,.F.);
#28057=ORIENTED_EDGE('',*,*,#20020,.F.);
#28058=ORIENTED_EDGE('',*,*,#19827,.F.);
#28059=ORIENTED_EDGE('',*,*,#20021,.F.);
#28060=ORIENTED_EDGE('',*,*,#20022,.F.);
#28061=ORIENTED_EDGE('',*,*,#20016,.T.);
#28062=ORIENTED_EDGE('',*,*,#19832,.F.);
#28063=ORIENTED_EDGE('',*,*,#20023,.F.);
#28064=ORIENTED_EDGE('',*,*,#20024,.F.);
#28065=ORIENTED_EDGE('',*,*,#20025,.T.);
#28066=ORIENTED_EDGE('',*,*,#19833,.F.);
#28067=ORIENTED_EDGE('',*,*,#20025,.F.);
#28068=ORIENTED_EDGE('',*,*,#20026,.F.);
#28069=ORIENTED_EDGE('',*,*,#20027,.F.);
#28070=ORIENTED_EDGE('',*,*,#19831,.F.);
#28071=ORIENTED_EDGE('',*,*,#20028,.F.);
#28072=ORIENTED_EDGE('',*,*,#20029,.F.);
#28073=ORIENTED_EDGE('',*,*,#20023,.T.);
#28074=ORIENTED_EDGE('',*,*,#19836,.F.);
#28075=ORIENTED_EDGE('',*,*,#20030,.F.);
#28076=ORIENTED_EDGE('',*,*,#20031,.F.);
#28077=ORIENTED_EDGE('',*,*,#20032,.T.);
#28078=ORIENTED_EDGE('',*,*,#19837,.F.);
#28079=ORIENTED_EDGE('',*,*,#20032,.F.);
#28080=ORIENTED_EDGE('',*,*,#20033,.F.);
#28081=ORIENTED_EDGE('',*,*,#20034,.F.);
#28082=ORIENTED_EDGE('',*,*,#19835,.F.);
#28083=ORIENTED_EDGE('',*,*,#20035,.F.);
#28084=ORIENTED_EDGE('',*,*,#20036,.F.);
#28085=ORIENTED_EDGE('',*,*,#20030,.T.);
#28086=ORIENTED_EDGE('',*,*,#19840,.F.);
#28087=ORIENTED_EDGE('',*,*,#20037,.F.);
#28088=ORIENTED_EDGE('',*,*,#20038,.F.);
#28089=ORIENTED_EDGE('',*,*,#20039,.T.);
#28090=ORIENTED_EDGE('',*,*,#19841,.F.);
#28091=ORIENTED_EDGE('',*,*,#20039,.F.);
#28092=ORIENTED_EDGE('',*,*,#20040,.F.);
#28093=ORIENTED_EDGE('',*,*,#20041,.F.);
#28094=ORIENTED_EDGE('',*,*,#19839,.F.);
#28095=ORIENTED_EDGE('',*,*,#20042,.F.);
#28096=ORIENTED_EDGE('',*,*,#20043,.F.);
#28097=ORIENTED_EDGE('',*,*,#20037,.T.);
#28098=ORIENTED_EDGE('',*,*,#19844,.F.);
#28099=ORIENTED_EDGE('',*,*,#20044,.F.);
#28100=ORIENTED_EDGE('',*,*,#20045,.F.);
#28101=ORIENTED_EDGE('',*,*,#20046,.T.);
#28102=ORIENTED_EDGE('',*,*,#19845,.F.);
#28103=ORIENTED_EDGE('',*,*,#20046,.F.);
#28104=ORIENTED_EDGE('',*,*,#20047,.F.);
#28105=ORIENTED_EDGE('',*,*,#20048,.F.);
#28106=ORIENTED_EDGE('',*,*,#19843,.F.);
#28107=ORIENTED_EDGE('',*,*,#20049,.F.);
#28108=ORIENTED_EDGE('',*,*,#20050,.F.);
#28109=ORIENTED_EDGE('',*,*,#20044,.T.);
#28110=ORIENTED_EDGE('',*,*,#19848,.F.);
#28111=ORIENTED_EDGE('',*,*,#20051,.F.);
#28112=ORIENTED_EDGE('',*,*,#20052,.F.);
#28113=ORIENTED_EDGE('',*,*,#20053,.T.);
#28114=ORIENTED_EDGE('',*,*,#19849,.F.);
#28115=ORIENTED_EDGE('',*,*,#20053,.F.);
#28116=ORIENTED_EDGE('',*,*,#20054,.F.);
#28117=ORIENTED_EDGE('',*,*,#20055,.F.);
#28118=ORIENTED_EDGE('',*,*,#19847,.F.);
#28119=ORIENTED_EDGE('',*,*,#20056,.F.);
#28120=ORIENTED_EDGE('',*,*,#20057,.F.);
#28121=ORIENTED_EDGE('',*,*,#20051,.T.);
#28122=ORIENTED_EDGE('',*,*,#19852,.F.);
#28123=ORIENTED_EDGE('',*,*,#20058,.F.);
#28124=ORIENTED_EDGE('',*,*,#20059,.F.);
#28125=ORIENTED_EDGE('',*,*,#20060,.T.);
#28126=ORIENTED_EDGE('',*,*,#19853,.F.);
#28127=ORIENTED_EDGE('',*,*,#20060,.F.);
#28128=ORIENTED_EDGE('',*,*,#20061,.F.);
#28129=ORIENTED_EDGE('',*,*,#20062,.F.);
#28130=ORIENTED_EDGE('',*,*,#19851,.F.);
#28131=ORIENTED_EDGE('',*,*,#20063,.F.);
#28132=ORIENTED_EDGE('',*,*,#20064,.F.);
#28133=ORIENTED_EDGE('',*,*,#20058,.T.);
#28134=ORIENTED_EDGE('',*,*,#19856,.F.);
#28135=ORIENTED_EDGE('',*,*,#20065,.F.);
#28136=ORIENTED_EDGE('',*,*,#20066,.F.);
#28137=ORIENTED_EDGE('',*,*,#20067,.T.);
#28138=ORIENTED_EDGE('',*,*,#19857,.F.);
#28139=ORIENTED_EDGE('',*,*,#20067,.F.);
#28140=ORIENTED_EDGE('',*,*,#20068,.F.);
#28141=ORIENTED_EDGE('',*,*,#20069,.F.);
#28142=ORIENTED_EDGE('',*,*,#19855,.F.);
#28143=ORIENTED_EDGE('',*,*,#20070,.F.);
#28144=ORIENTED_EDGE('',*,*,#20071,.F.);
#28145=ORIENTED_EDGE('',*,*,#20065,.T.);
#28146=ORIENTED_EDGE('',*,*,#19860,.F.);
#28147=ORIENTED_EDGE('',*,*,#20072,.F.);
#28148=ORIENTED_EDGE('',*,*,#20073,.F.);
#28149=ORIENTED_EDGE('',*,*,#20074,.T.);
#28150=ORIENTED_EDGE('',*,*,#19861,.F.);
#28151=ORIENTED_EDGE('',*,*,#20074,.F.);
#28152=ORIENTED_EDGE('',*,*,#20075,.F.);
#28153=ORIENTED_EDGE('',*,*,#20076,.F.);
#28154=ORIENTED_EDGE('',*,*,#19859,.F.);
#28155=ORIENTED_EDGE('',*,*,#20077,.F.);
#28156=ORIENTED_EDGE('',*,*,#20078,.F.);
#28157=ORIENTED_EDGE('',*,*,#20072,.T.);
#28158=ORIENTED_EDGE('',*,*,#19864,.F.);
#28159=ORIENTED_EDGE('',*,*,#20079,.F.);
#28160=ORIENTED_EDGE('',*,*,#20080,.F.);
#28161=ORIENTED_EDGE('',*,*,#20081,.T.);
#28162=ORIENTED_EDGE('',*,*,#19865,.F.);
#28163=ORIENTED_EDGE('',*,*,#20081,.F.);
#28164=ORIENTED_EDGE('',*,*,#20082,.F.);
#28165=ORIENTED_EDGE('',*,*,#20083,.F.);
#28166=ORIENTED_EDGE('',*,*,#19863,.F.);
#28167=ORIENTED_EDGE('',*,*,#20084,.F.);
#28168=ORIENTED_EDGE('',*,*,#20085,.F.);
#28169=ORIENTED_EDGE('',*,*,#20079,.T.);
#28170=ORIENTED_EDGE('',*,*,#19868,.F.);
#28171=ORIENTED_EDGE('',*,*,#20086,.F.);
#28172=ORIENTED_EDGE('',*,*,#20087,.F.);
#28173=ORIENTED_EDGE('',*,*,#20088,.T.);
#28174=ORIENTED_EDGE('',*,*,#19869,.F.);
#28175=ORIENTED_EDGE('',*,*,#20088,.F.);
#28176=ORIENTED_EDGE('',*,*,#20089,.F.);
#28177=ORIENTED_EDGE('',*,*,#20090,.F.);
#28178=ORIENTED_EDGE('',*,*,#19867,.F.);
#28179=ORIENTED_EDGE('',*,*,#20091,.F.);
#28180=ORIENTED_EDGE('',*,*,#20092,.F.);
#28181=ORIENTED_EDGE('',*,*,#20086,.T.);
#28182=ORIENTED_EDGE('',*,*,#19872,.F.);
#28183=ORIENTED_EDGE('',*,*,#20093,.F.);
#28184=ORIENTED_EDGE('',*,*,#20094,.F.);
#28185=ORIENTED_EDGE('',*,*,#20095,.T.);
#28186=ORIENTED_EDGE('',*,*,#19873,.F.);
#28187=ORIENTED_EDGE('',*,*,#20095,.F.);
#28188=ORIENTED_EDGE('',*,*,#20096,.F.);
#28189=ORIENTED_EDGE('',*,*,#20097,.F.);
#28190=ORIENTED_EDGE('',*,*,#19871,.F.);
#28191=ORIENTED_EDGE('',*,*,#20098,.F.);
#28192=ORIENTED_EDGE('',*,*,#20099,.F.);
#28193=ORIENTED_EDGE('',*,*,#20093,.T.);
#28194=ORIENTED_EDGE('',*,*,#19876,.F.);
#28195=ORIENTED_EDGE('',*,*,#20100,.F.);
#28196=ORIENTED_EDGE('',*,*,#20101,.F.);
#28197=ORIENTED_EDGE('',*,*,#20102,.T.);
#28198=ORIENTED_EDGE('',*,*,#19877,.F.);
#28199=ORIENTED_EDGE('',*,*,#20102,.F.);
#28200=ORIENTED_EDGE('',*,*,#20103,.F.);
#28201=ORIENTED_EDGE('',*,*,#20104,.F.);
#28202=ORIENTED_EDGE('',*,*,#19875,.F.);
#28203=ORIENTED_EDGE('',*,*,#20105,.F.);
#28204=ORIENTED_EDGE('',*,*,#20106,.F.);
#28205=ORIENTED_EDGE('',*,*,#20100,.T.);
#28206=ORIENTED_EDGE('',*,*,#19880,.F.);
#28207=ORIENTED_EDGE('',*,*,#20107,.F.);
#28208=ORIENTED_EDGE('',*,*,#20108,.F.);
#28209=ORIENTED_EDGE('',*,*,#20109,.T.);
#28210=ORIENTED_EDGE('',*,*,#19881,.F.);
#28211=ORIENTED_EDGE('',*,*,#20109,.F.);
#28212=ORIENTED_EDGE('',*,*,#20110,.F.);
#28213=ORIENTED_EDGE('',*,*,#20111,.F.);
#28214=ORIENTED_EDGE('',*,*,#19879,.F.);
#28215=ORIENTED_EDGE('',*,*,#20112,.F.);
#28216=ORIENTED_EDGE('',*,*,#20113,.F.);
#28217=ORIENTED_EDGE('',*,*,#20107,.T.);
#28218=ORIENTED_EDGE('',*,*,#19884,.F.);
#28219=ORIENTED_EDGE('',*,*,#20114,.F.);
#28220=ORIENTED_EDGE('',*,*,#20115,.F.);
#28221=ORIENTED_EDGE('',*,*,#20116,.T.);
#28222=ORIENTED_EDGE('',*,*,#19885,.F.);
#28223=ORIENTED_EDGE('',*,*,#20116,.F.);
#28224=ORIENTED_EDGE('',*,*,#20117,.F.);
#28225=ORIENTED_EDGE('',*,*,#20118,.F.);
#28226=ORIENTED_EDGE('',*,*,#19883,.F.);
#28227=ORIENTED_EDGE('',*,*,#20119,.F.);
#28228=ORIENTED_EDGE('',*,*,#20120,.F.);
#28229=ORIENTED_EDGE('',*,*,#20114,.T.);
#28230=ORIENTED_EDGE('',*,*,#19888,.F.);
#28231=ORIENTED_EDGE('',*,*,#20121,.F.);
#28232=ORIENTED_EDGE('',*,*,#20122,.F.);
#28233=ORIENTED_EDGE('',*,*,#20123,.T.);
#28234=ORIENTED_EDGE('',*,*,#19889,.F.);
#28235=ORIENTED_EDGE('',*,*,#20123,.F.);
#28236=ORIENTED_EDGE('',*,*,#20124,.F.);
#28237=ORIENTED_EDGE('',*,*,#20125,.F.);
#28238=ORIENTED_EDGE('',*,*,#19887,.F.);
#28239=ORIENTED_EDGE('',*,*,#20126,.F.);
#28240=ORIENTED_EDGE('',*,*,#20127,.F.);
#28241=ORIENTED_EDGE('',*,*,#20121,.T.);
#28242=ORIENTED_EDGE('',*,*,#19892,.F.);
#28243=ORIENTED_EDGE('',*,*,#20128,.F.);
#28244=ORIENTED_EDGE('',*,*,#20129,.F.);
#28245=ORIENTED_EDGE('',*,*,#20130,.T.);
#28246=ORIENTED_EDGE('',*,*,#19893,.F.);
#28247=ORIENTED_EDGE('',*,*,#20130,.F.);
#28248=ORIENTED_EDGE('',*,*,#20131,.F.);
#28249=ORIENTED_EDGE('',*,*,#20132,.F.);
#28250=ORIENTED_EDGE('',*,*,#19891,.F.);
#28251=ORIENTED_EDGE('',*,*,#20133,.F.);
#28252=ORIENTED_EDGE('',*,*,#20134,.F.);
#28253=ORIENTED_EDGE('',*,*,#20128,.T.);
#28254=ORIENTED_EDGE('',*,*,#19896,.F.);
#28255=ORIENTED_EDGE('',*,*,#20135,.F.);
#28256=ORIENTED_EDGE('',*,*,#20136,.F.);
#28257=ORIENTED_EDGE('',*,*,#20137,.T.);
#28258=ORIENTED_EDGE('',*,*,#19897,.F.);
#28259=ORIENTED_EDGE('',*,*,#20137,.F.);
#28260=ORIENTED_EDGE('',*,*,#20138,.F.);
#28261=ORIENTED_EDGE('',*,*,#20139,.F.);
#28262=ORIENTED_EDGE('',*,*,#19895,.F.);
#28263=ORIENTED_EDGE('',*,*,#20140,.F.);
#28264=ORIENTED_EDGE('',*,*,#20141,.F.);
#28265=ORIENTED_EDGE('',*,*,#20135,.T.);
#28266=ORIENTED_EDGE('',*,*,#19900,.F.);
#28267=ORIENTED_EDGE('',*,*,#20142,.F.);
#28268=ORIENTED_EDGE('',*,*,#20143,.F.);
#28269=ORIENTED_EDGE('',*,*,#20144,.T.);
#28270=ORIENTED_EDGE('',*,*,#19901,.F.);
#28271=ORIENTED_EDGE('',*,*,#20144,.F.);
#28272=ORIENTED_EDGE('',*,*,#20145,.F.);
#28273=ORIENTED_EDGE('',*,*,#20146,.F.);
#28274=ORIENTED_EDGE('',*,*,#19899,.F.);
#28275=ORIENTED_EDGE('',*,*,#20147,.F.);
#28276=ORIENTED_EDGE('',*,*,#20148,.F.);
#28277=ORIENTED_EDGE('',*,*,#20142,.T.);
#28278=ORIENTED_EDGE('',*,*,#19904,.F.);
#28279=ORIENTED_EDGE('',*,*,#20149,.F.);
#28280=ORIENTED_EDGE('',*,*,#20150,.F.);
#28281=ORIENTED_EDGE('',*,*,#20151,.T.);
#28282=ORIENTED_EDGE('',*,*,#19905,.F.);
#28283=ORIENTED_EDGE('',*,*,#20151,.F.);
#28284=ORIENTED_EDGE('',*,*,#20152,.F.);
#28285=ORIENTED_EDGE('',*,*,#20153,.F.);
#28286=ORIENTED_EDGE('',*,*,#19903,.F.);
#28287=ORIENTED_EDGE('',*,*,#20154,.F.);
#28288=ORIENTED_EDGE('',*,*,#20155,.F.);
#28289=ORIENTED_EDGE('',*,*,#20149,.T.);
#28290=ORIENTED_EDGE('',*,*,#19908,.F.);
#28291=ORIENTED_EDGE('',*,*,#20156,.F.);
#28292=ORIENTED_EDGE('',*,*,#20157,.F.);
#28293=ORIENTED_EDGE('',*,*,#20158,.T.);
#28294=ORIENTED_EDGE('',*,*,#19909,.F.);
#28295=ORIENTED_EDGE('',*,*,#20158,.F.);
#28296=ORIENTED_EDGE('',*,*,#20159,.F.);
#28297=ORIENTED_EDGE('',*,*,#20160,.F.);
#28298=ORIENTED_EDGE('',*,*,#19907,.F.);
#28299=ORIENTED_EDGE('',*,*,#20161,.F.);
#28300=ORIENTED_EDGE('',*,*,#20162,.F.);
#28301=ORIENTED_EDGE('',*,*,#20156,.T.);
#28302=ORIENTED_EDGE('',*,*,#19912,.F.);
#28303=ORIENTED_EDGE('',*,*,#20163,.F.);
#28304=ORIENTED_EDGE('',*,*,#20164,.F.);
#28305=ORIENTED_EDGE('',*,*,#20165,.T.);
#28306=ORIENTED_EDGE('',*,*,#19913,.F.);
#28307=ORIENTED_EDGE('',*,*,#20165,.F.);
#28308=ORIENTED_EDGE('',*,*,#20166,.F.);
#28309=ORIENTED_EDGE('',*,*,#20167,.F.);
#28310=ORIENTED_EDGE('',*,*,#19911,.F.);
#28311=ORIENTED_EDGE('',*,*,#20168,.F.);
#28312=ORIENTED_EDGE('',*,*,#20169,.F.);
#28313=ORIENTED_EDGE('',*,*,#20163,.T.);
#28314=ORIENTED_EDGE('',*,*,#19916,.F.);
#28315=ORIENTED_EDGE('',*,*,#20170,.F.);
#28316=ORIENTED_EDGE('',*,*,#20171,.F.);
#28317=ORIENTED_EDGE('',*,*,#20172,.T.);
#28318=ORIENTED_EDGE('',*,*,#19917,.F.);
#28319=ORIENTED_EDGE('',*,*,#20172,.F.);
#28320=ORIENTED_EDGE('',*,*,#20173,.F.);
#28321=ORIENTED_EDGE('',*,*,#20174,.F.);
#28322=ORIENTED_EDGE('',*,*,#19915,.F.);
#28323=ORIENTED_EDGE('',*,*,#20175,.F.);
#28324=ORIENTED_EDGE('',*,*,#20176,.F.);
#28325=ORIENTED_EDGE('',*,*,#20170,.T.);
#28326=ORIENTED_EDGE('',*,*,#19920,.F.);
#28327=ORIENTED_EDGE('',*,*,#20177,.F.);
#28328=ORIENTED_EDGE('',*,*,#20178,.F.);
#28329=ORIENTED_EDGE('',*,*,#20179,.T.);
#28330=ORIENTED_EDGE('',*,*,#19921,.F.);
#28331=ORIENTED_EDGE('',*,*,#20179,.F.);
#28332=ORIENTED_EDGE('',*,*,#20180,.F.);
#28333=ORIENTED_EDGE('',*,*,#20181,.F.);
#28334=ORIENTED_EDGE('',*,*,#19919,.F.);
#28335=ORIENTED_EDGE('',*,*,#20182,.F.);
#28336=ORIENTED_EDGE('',*,*,#20183,.F.);
#28337=ORIENTED_EDGE('',*,*,#20177,.T.);
#28338=ORIENTED_EDGE('',*,*,#19924,.F.);
#28339=ORIENTED_EDGE('',*,*,#20184,.F.);
#28340=ORIENTED_EDGE('',*,*,#20185,.F.);
#28341=ORIENTED_EDGE('',*,*,#20186,.T.);
#28342=ORIENTED_EDGE('',*,*,#19925,.F.);
#28343=ORIENTED_EDGE('',*,*,#20186,.F.);
#28344=ORIENTED_EDGE('',*,*,#20187,.F.);
#28345=ORIENTED_EDGE('',*,*,#20188,.F.);
#28346=ORIENTED_EDGE('',*,*,#19923,.F.);
#28347=ORIENTED_EDGE('',*,*,#20189,.F.);
#28348=ORIENTED_EDGE('',*,*,#20190,.F.);
#28349=ORIENTED_EDGE('',*,*,#20184,.T.);
#28350=ORIENTED_EDGE('',*,*,#19928,.F.);
#28351=ORIENTED_EDGE('',*,*,#20191,.F.);
#28352=ORIENTED_EDGE('',*,*,#20192,.F.);
#28353=ORIENTED_EDGE('',*,*,#20193,.T.);
#28354=ORIENTED_EDGE('',*,*,#19929,.F.);
#28355=ORIENTED_EDGE('',*,*,#20193,.F.);
#28356=ORIENTED_EDGE('',*,*,#20194,.F.);
#28357=ORIENTED_EDGE('',*,*,#20195,.F.);
#28358=ORIENTED_EDGE('',*,*,#19927,.F.);
#28359=ORIENTED_EDGE('',*,*,#20196,.F.);
#28360=ORIENTED_EDGE('',*,*,#20197,.F.);
#28361=ORIENTED_EDGE('',*,*,#20191,.T.);
#28362=ORIENTED_EDGE('',*,*,#19932,.F.);
#28363=ORIENTED_EDGE('',*,*,#20198,.F.);
#28364=ORIENTED_EDGE('',*,*,#20199,.F.);
#28365=ORIENTED_EDGE('',*,*,#20200,.T.);
#28366=ORIENTED_EDGE('',*,*,#19933,.F.);
#28367=ORIENTED_EDGE('',*,*,#20200,.F.);
#28368=ORIENTED_EDGE('',*,*,#20201,.F.);
#28369=ORIENTED_EDGE('',*,*,#20202,.F.);
#28370=ORIENTED_EDGE('',*,*,#19931,.F.);
#28371=ORIENTED_EDGE('',*,*,#20203,.F.);
#28372=ORIENTED_EDGE('',*,*,#20204,.F.);
#28373=ORIENTED_EDGE('',*,*,#20198,.T.);
#28374=ORIENTED_EDGE('',*,*,#19936,.F.);
#28375=ORIENTED_EDGE('',*,*,#20205,.F.);
#28376=ORIENTED_EDGE('',*,*,#20206,.F.);
#28377=ORIENTED_EDGE('',*,*,#20207,.T.);
#28378=ORIENTED_EDGE('',*,*,#19937,.F.);
#28379=ORIENTED_EDGE('',*,*,#20207,.F.);
#28380=ORIENTED_EDGE('',*,*,#20208,.F.);
#28381=ORIENTED_EDGE('',*,*,#20209,.F.);
#28382=ORIENTED_EDGE('',*,*,#19935,.F.);
#28383=ORIENTED_EDGE('',*,*,#20210,.F.);
#28384=ORIENTED_EDGE('',*,*,#20211,.F.);
#28385=ORIENTED_EDGE('',*,*,#20205,.T.);
#28386=ORIENTED_EDGE('',*,*,#19940,.F.);
#28387=ORIENTED_EDGE('',*,*,#20212,.F.);
#28388=ORIENTED_EDGE('',*,*,#20213,.F.);
#28389=ORIENTED_EDGE('',*,*,#20214,.T.);
#28390=ORIENTED_EDGE('',*,*,#19941,.F.);
#28391=ORIENTED_EDGE('',*,*,#20214,.F.);
#28392=ORIENTED_EDGE('',*,*,#20215,.F.);
#28393=ORIENTED_EDGE('',*,*,#20216,.F.);
#28394=ORIENTED_EDGE('',*,*,#19939,.F.);
#28395=ORIENTED_EDGE('',*,*,#20217,.F.);
#28396=ORIENTED_EDGE('',*,*,#20218,.F.);
#28397=ORIENTED_EDGE('',*,*,#20212,.T.);
#28398=ORIENTED_EDGE('',*,*,#19944,.F.);
#28399=ORIENTED_EDGE('',*,*,#20219,.F.);
#28400=ORIENTED_EDGE('',*,*,#20220,.F.);
#28401=ORIENTED_EDGE('',*,*,#20221,.T.);
#28402=ORIENTED_EDGE('',*,*,#19945,.F.);
#28403=ORIENTED_EDGE('',*,*,#20221,.F.);
#28404=ORIENTED_EDGE('',*,*,#20222,.F.);
#28405=ORIENTED_EDGE('',*,*,#20223,.F.);
#28406=ORIENTED_EDGE('',*,*,#19943,.F.);
#28407=ORIENTED_EDGE('',*,*,#20224,.F.);
#28408=ORIENTED_EDGE('',*,*,#20225,.F.);
#28409=ORIENTED_EDGE('',*,*,#20219,.T.);
#28410=ORIENTED_EDGE('',*,*,#19948,.F.);
#28411=ORIENTED_EDGE('',*,*,#20226,.F.);
#28412=ORIENTED_EDGE('',*,*,#20227,.F.);
#28413=ORIENTED_EDGE('',*,*,#20228,.T.);
#28414=ORIENTED_EDGE('',*,*,#19949,.F.);
#28415=ORIENTED_EDGE('',*,*,#20228,.F.);
#28416=ORIENTED_EDGE('',*,*,#20229,.F.);
#28417=ORIENTED_EDGE('',*,*,#20230,.F.);
#28418=ORIENTED_EDGE('',*,*,#19947,.F.);
#28419=ORIENTED_EDGE('',*,*,#20231,.F.);
#28420=ORIENTED_EDGE('',*,*,#20232,.F.);
#28421=ORIENTED_EDGE('',*,*,#20226,.T.);
#28422=ORIENTED_EDGE('',*,*,#19952,.F.);
#28423=ORIENTED_EDGE('',*,*,#20233,.F.);
#28424=ORIENTED_EDGE('',*,*,#20234,.F.);
#28425=ORIENTED_EDGE('',*,*,#20235,.T.);
#28426=ORIENTED_EDGE('',*,*,#19953,.F.);
#28427=ORIENTED_EDGE('',*,*,#20235,.F.);
#28428=ORIENTED_EDGE('',*,*,#20236,.F.);
#28429=ORIENTED_EDGE('',*,*,#20237,.F.);
#28430=ORIENTED_EDGE('',*,*,#19951,.F.);
#28431=ORIENTED_EDGE('',*,*,#20238,.F.);
#28432=ORIENTED_EDGE('',*,*,#20239,.F.);
#28433=ORIENTED_EDGE('',*,*,#20233,.T.);
#28434=ORIENTED_EDGE('',*,*,#20237,.T.);
#28435=ORIENTED_EDGE('',*,*,#20240,.F.);
#28436=ORIENTED_EDGE('',*,*,#20241,.T.);
#28437=ORIENTED_EDGE('',*,*,#19954,.T.);
#28438=ORIENTED_EDGE('',*,*,#20230,.T.);
#28439=ORIENTED_EDGE('',*,*,#20242,.F.);
#28440=ORIENTED_EDGE('',*,*,#20238,.T.);
#28441=ORIENTED_EDGE('',*,*,#19950,.T.);
#28442=ORIENTED_EDGE('',*,*,#20223,.T.);
#28443=ORIENTED_EDGE('',*,*,#20243,.F.);
#28444=ORIENTED_EDGE('',*,*,#20231,.T.);
#28445=ORIENTED_EDGE('',*,*,#19946,.T.);
#28446=ORIENTED_EDGE('',*,*,#20216,.T.);
#28447=ORIENTED_EDGE('',*,*,#20244,.F.);
#28448=ORIENTED_EDGE('',*,*,#20224,.T.);
#28449=ORIENTED_EDGE('',*,*,#19942,.T.);
#28450=ORIENTED_EDGE('',*,*,#20209,.T.);
#28451=ORIENTED_EDGE('',*,*,#20245,.F.);
#28452=ORIENTED_EDGE('',*,*,#20217,.T.);
#28453=ORIENTED_EDGE('',*,*,#19938,.T.);
#28454=ORIENTED_EDGE('',*,*,#20202,.T.);
#28455=ORIENTED_EDGE('',*,*,#20246,.F.);
#28456=ORIENTED_EDGE('',*,*,#20210,.T.);
#28457=ORIENTED_EDGE('',*,*,#19934,.T.);
#28458=ORIENTED_EDGE('',*,*,#20195,.T.);
#28459=ORIENTED_EDGE('',*,*,#20247,.F.);
#28460=ORIENTED_EDGE('',*,*,#20203,.T.);
#28461=ORIENTED_EDGE('',*,*,#19930,.T.);
#28462=ORIENTED_EDGE('',*,*,#20188,.T.);
#28463=ORIENTED_EDGE('',*,*,#20248,.F.);
#28464=ORIENTED_EDGE('',*,*,#20196,.T.);
#28465=ORIENTED_EDGE('',*,*,#19926,.T.);
#28466=ORIENTED_EDGE('',*,*,#20181,.T.);
#28467=ORIENTED_EDGE('',*,*,#20249,.F.);
#28468=ORIENTED_EDGE('',*,*,#20189,.T.);
#28469=ORIENTED_EDGE('',*,*,#19922,.T.);
#28470=ORIENTED_EDGE('',*,*,#20174,.T.);
#28471=ORIENTED_EDGE('',*,*,#20250,.F.);
#28472=ORIENTED_EDGE('',*,*,#20182,.T.);
#28473=ORIENTED_EDGE('',*,*,#19918,.T.);
#28474=ORIENTED_EDGE('',*,*,#20167,.T.);
#28475=ORIENTED_EDGE('',*,*,#20251,.F.);
#28476=ORIENTED_EDGE('',*,*,#20175,.T.);
#28477=ORIENTED_EDGE('',*,*,#19914,.T.);
#28478=ORIENTED_EDGE('',*,*,#20160,.T.);
#28479=ORIENTED_EDGE('',*,*,#20252,.F.);
#28480=ORIENTED_EDGE('',*,*,#20168,.T.);
#28481=ORIENTED_EDGE('',*,*,#19910,.T.);
#28482=ORIENTED_EDGE('',*,*,#20153,.T.);
#28483=ORIENTED_EDGE('',*,*,#20253,.F.);
#28484=ORIENTED_EDGE('',*,*,#20161,.T.);
#28485=ORIENTED_EDGE('',*,*,#19906,.T.);
#28486=ORIENTED_EDGE('',*,*,#20146,.T.);
#28487=ORIENTED_EDGE('',*,*,#20254,.F.);
#28488=ORIENTED_EDGE('',*,*,#20154,.T.);
#28489=ORIENTED_EDGE('',*,*,#19902,.T.);
#28490=ORIENTED_EDGE('',*,*,#20139,.T.);
#28491=ORIENTED_EDGE('',*,*,#20255,.F.);
#28492=ORIENTED_EDGE('',*,*,#20147,.T.);
#28493=ORIENTED_EDGE('',*,*,#19898,.T.);
#28494=ORIENTED_EDGE('',*,*,#20132,.T.);
#28495=ORIENTED_EDGE('',*,*,#20256,.F.);
#28496=ORIENTED_EDGE('',*,*,#20140,.T.);
#28497=ORIENTED_EDGE('',*,*,#19894,.T.);
#28498=ORIENTED_EDGE('',*,*,#20125,.T.);
#28499=ORIENTED_EDGE('',*,*,#20257,.F.);
#28500=ORIENTED_EDGE('',*,*,#20133,.T.);
#28501=ORIENTED_EDGE('',*,*,#19890,.T.);
#28502=ORIENTED_EDGE('',*,*,#20118,.T.);
#28503=ORIENTED_EDGE('',*,*,#20258,.F.);
#28504=ORIENTED_EDGE('',*,*,#20126,.T.);
#28505=ORIENTED_EDGE('',*,*,#19886,.T.);
#28506=ORIENTED_EDGE('',*,*,#20111,.T.);
#28507=ORIENTED_EDGE('',*,*,#20259,.F.);
#28508=ORIENTED_EDGE('',*,*,#20119,.T.);
#28509=ORIENTED_EDGE('',*,*,#19882,.T.);
#28510=ORIENTED_EDGE('',*,*,#20104,.T.);
#28511=ORIENTED_EDGE('',*,*,#20260,.F.);
#28512=ORIENTED_EDGE('',*,*,#20112,.T.);
#28513=ORIENTED_EDGE('',*,*,#19878,.T.);
#28514=ORIENTED_EDGE('',*,*,#20097,.T.);
#28515=ORIENTED_EDGE('',*,*,#20261,.F.);
#28516=ORIENTED_EDGE('',*,*,#20105,.T.);
#28517=ORIENTED_EDGE('',*,*,#19874,.T.);
#28518=ORIENTED_EDGE('',*,*,#20090,.T.);
#28519=ORIENTED_EDGE('',*,*,#20262,.F.);
#28520=ORIENTED_EDGE('',*,*,#20098,.T.);
#28521=ORIENTED_EDGE('',*,*,#19870,.T.);
#28522=ORIENTED_EDGE('',*,*,#20083,.T.);
#28523=ORIENTED_EDGE('',*,*,#20263,.F.);
#28524=ORIENTED_EDGE('',*,*,#20091,.T.);
#28525=ORIENTED_EDGE('',*,*,#19866,.T.);
#28526=ORIENTED_EDGE('',*,*,#20076,.T.);
#28527=ORIENTED_EDGE('',*,*,#20264,.F.);
#28528=ORIENTED_EDGE('',*,*,#20084,.T.);
#28529=ORIENTED_EDGE('',*,*,#19862,.T.);
#28530=ORIENTED_EDGE('',*,*,#20069,.T.);
#28531=ORIENTED_EDGE('',*,*,#20265,.F.);
#28532=ORIENTED_EDGE('',*,*,#20077,.T.);
#28533=ORIENTED_EDGE('',*,*,#19858,.T.);
#28534=ORIENTED_EDGE('',*,*,#20062,.T.);
#28535=ORIENTED_EDGE('',*,*,#20266,.F.);
#28536=ORIENTED_EDGE('',*,*,#20070,.T.);
#28537=ORIENTED_EDGE('',*,*,#19854,.T.);
#28538=ORIENTED_EDGE('',*,*,#20055,.T.);
#28539=ORIENTED_EDGE('',*,*,#20267,.F.);
#28540=ORIENTED_EDGE('',*,*,#20063,.T.);
#28541=ORIENTED_EDGE('',*,*,#19850,.T.);
#28542=ORIENTED_EDGE('',*,*,#20048,.T.);
#28543=ORIENTED_EDGE('',*,*,#20268,.F.);
#28544=ORIENTED_EDGE('',*,*,#20056,.T.);
#28545=ORIENTED_EDGE('',*,*,#19846,.T.);
#28546=ORIENTED_EDGE('',*,*,#20041,.T.);
#28547=ORIENTED_EDGE('',*,*,#20269,.F.);
#28548=ORIENTED_EDGE('',*,*,#20049,.T.);
#28549=ORIENTED_EDGE('',*,*,#19842,.T.);
#28550=ORIENTED_EDGE('',*,*,#20034,.T.);
#28551=ORIENTED_EDGE('',*,*,#20270,.F.);
#28552=ORIENTED_EDGE('',*,*,#20042,.T.);
#28553=ORIENTED_EDGE('',*,*,#19838,.T.);
#28554=ORIENTED_EDGE('',*,*,#20027,.T.);
#28555=ORIENTED_EDGE('',*,*,#20271,.F.);
#28556=ORIENTED_EDGE('',*,*,#20035,.T.);
#28557=ORIENTED_EDGE('',*,*,#19834,.T.);
#28558=ORIENTED_EDGE('',*,*,#20020,.T.);
#28559=ORIENTED_EDGE('',*,*,#20272,.F.);
#28560=ORIENTED_EDGE('',*,*,#20028,.T.);
#28561=ORIENTED_EDGE('',*,*,#19830,.T.);
#28562=ORIENTED_EDGE('',*,*,#20013,.T.);
#28563=ORIENTED_EDGE('',*,*,#20273,.F.);
#28564=ORIENTED_EDGE('',*,*,#20021,.T.);
#28565=ORIENTED_EDGE('',*,*,#19826,.T.);
#28566=ORIENTED_EDGE('',*,*,#20006,.T.);
#28567=ORIENTED_EDGE('',*,*,#20274,.F.);
#28568=ORIENTED_EDGE('',*,*,#20014,.T.);
#28569=ORIENTED_EDGE('',*,*,#19822,.T.);
#28570=ORIENTED_EDGE('',*,*,#19999,.T.);
#28571=ORIENTED_EDGE('',*,*,#20275,.F.);
#28572=ORIENTED_EDGE('',*,*,#20007,.T.);
#28573=ORIENTED_EDGE('',*,*,#19818,.T.);
#28574=ORIENTED_EDGE('',*,*,#19992,.T.);
#28575=ORIENTED_EDGE('',*,*,#20276,.F.);
#28576=ORIENTED_EDGE('',*,*,#20000,.T.);
#28577=ORIENTED_EDGE('',*,*,#19814,.T.);
#28578=ORIENTED_EDGE('',*,*,#19985,.T.);
#28579=ORIENTED_EDGE('',*,*,#20277,.F.);
#28580=ORIENTED_EDGE('',*,*,#19993,.T.);
#28581=ORIENTED_EDGE('',*,*,#19810,.T.);
#28582=ORIENTED_EDGE('',*,*,#19978,.T.);
#28583=ORIENTED_EDGE('',*,*,#20278,.F.);
#28584=ORIENTED_EDGE('',*,*,#19986,.T.);
#28585=ORIENTED_EDGE('',*,*,#19806,.T.);
#28586=ORIENTED_EDGE('',*,*,#19971,.T.);
#28587=ORIENTED_EDGE('',*,*,#20279,.F.);
#28588=ORIENTED_EDGE('',*,*,#19979,.T.);
#28589=ORIENTED_EDGE('',*,*,#19802,.T.);
#28590=ORIENTED_EDGE('',*,*,#19956,.F.);
#28591=ORIENTED_EDGE('',*,*,#20280,.F.);
#28592=ORIENTED_EDGE('',*,*,#20281,.F.);
#28593=ORIENTED_EDGE('',*,*,#20282,.T.);
#28594=ORIENTED_EDGE('',*,*,#19957,.F.);
#28595=ORIENTED_EDGE('',*,*,#20282,.F.);
#28596=ORIENTED_EDGE('',*,*,#20283,.F.);
#28597=ORIENTED_EDGE('',*,*,#20284,.F.);
#28598=ORIENTED_EDGE('',*,*,#19955,.F.);
#28599=ORIENTED_EDGE('',*,*,#20241,.F.);
#28600=ORIENTED_EDGE('',*,*,#20285,.F.);
#28601=ORIENTED_EDGE('',*,*,#20280,.T.);
#28602=ORIENTED_EDGE('',*,*,#19972,.T.);
#28603=ORIENTED_EDGE('',*,*,#19958,.T.);
#28604=ORIENTED_EDGE('',*,*,#20284,.T.);
#28605=ORIENTED_EDGE('',*,*,#20286,.F.);
#28606=ORIENTED_EDGE('',*,*,#19973,.T.);
#28607=ORIENTED_EDGE('',*,*,#20286,.T.);
#28608=ORIENTED_EDGE('',*,*,#20283,.T.);
#28609=ORIENTED_EDGE('',*,*,#20281,.T.);
#28610=ORIENTED_EDGE('',*,*,#20285,.T.);
#28611=ORIENTED_EDGE('',*,*,#20240,.T.);
#28612=ORIENTED_EDGE('',*,*,#20236,.T.);
#28613=ORIENTED_EDGE('',*,*,#20234,.T.);
#28614=ORIENTED_EDGE('',*,*,#20239,.T.);
#28615=ORIENTED_EDGE('',*,*,#20242,.T.);
#28616=ORIENTED_EDGE('',*,*,#20229,.T.);
#28617=ORIENTED_EDGE('',*,*,#20227,.T.);
#28618=ORIENTED_EDGE('',*,*,#20232,.T.);
#28619=ORIENTED_EDGE('',*,*,#20243,.T.);
#28620=ORIENTED_EDGE('',*,*,#20222,.T.);
#28621=ORIENTED_EDGE('',*,*,#20220,.T.);
#28622=ORIENTED_EDGE('',*,*,#20225,.T.);
#28623=ORIENTED_EDGE('',*,*,#20244,.T.);
#28624=ORIENTED_EDGE('',*,*,#20215,.T.);
#28625=ORIENTED_EDGE('',*,*,#20213,.T.);
#28626=ORIENTED_EDGE('',*,*,#20218,.T.);
#28627=ORIENTED_EDGE('',*,*,#20245,.T.);
#28628=ORIENTED_EDGE('',*,*,#20208,.T.);
#28629=ORIENTED_EDGE('',*,*,#20206,.T.);
#28630=ORIENTED_EDGE('',*,*,#20211,.T.);
#28631=ORIENTED_EDGE('',*,*,#20246,.T.);
#28632=ORIENTED_EDGE('',*,*,#20201,.T.);
#28633=ORIENTED_EDGE('',*,*,#20199,.T.);
#28634=ORIENTED_EDGE('',*,*,#20204,.T.);
#28635=ORIENTED_EDGE('',*,*,#20247,.T.);
#28636=ORIENTED_EDGE('',*,*,#20194,.T.);
#28637=ORIENTED_EDGE('',*,*,#20192,.T.);
#28638=ORIENTED_EDGE('',*,*,#20197,.T.);
#28639=ORIENTED_EDGE('',*,*,#20248,.T.);
#28640=ORIENTED_EDGE('',*,*,#20187,.T.);
#28641=ORIENTED_EDGE('',*,*,#20185,.T.);
#28642=ORIENTED_EDGE('',*,*,#20190,.T.);
#28643=ORIENTED_EDGE('',*,*,#20249,.T.);
#28644=ORIENTED_EDGE('',*,*,#20180,.T.);
#28645=ORIENTED_EDGE('',*,*,#20178,.T.);
#28646=ORIENTED_EDGE('',*,*,#20183,.T.);
#28647=ORIENTED_EDGE('',*,*,#20250,.T.);
#28648=ORIENTED_EDGE('',*,*,#20173,.T.);
#28649=ORIENTED_EDGE('',*,*,#20171,.T.);
#28650=ORIENTED_EDGE('',*,*,#20176,.T.);
#28651=ORIENTED_EDGE('',*,*,#20251,.T.);
#28652=ORIENTED_EDGE('',*,*,#20166,.T.);
#28653=ORIENTED_EDGE('',*,*,#20164,.T.);
#28654=ORIENTED_EDGE('',*,*,#20169,.T.);
#28655=ORIENTED_EDGE('',*,*,#20252,.T.);
#28656=ORIENTED_EDGE('',*,*,#20159,.T.);
#28657=ORIENTED_EDGE('',*,*,#20157,.T.);
#28658=ORIENTED_EDGE('',*,*,#20162,.T.);
#28659=ORIENTED_EDGE('',*,*,#20253,.T.);
#28660=ORIENTED_EDGE('',*,*,#20152,.T.);
#28661=ORIENTED_EDGE('',*,*,#20150,.T.);
#28662=ORIENTED_EDGE('',*,*,#20155,.T.);
#28663=ORIENTED_EDGE('',*,*,#20254,.T.);
#28664=ORIENTED_EDGE('',*,*,#20145,.T.);
#28665=ORIENTED_EDGE('',*,*,#20143,.T.);
#28666=ORIENTED_EDGE('',*,*,#20148,.T.);
#28667=ORIENTED_EDGE('',*,*,#20255,.T.);
#28668=ORIENTED_EDGE('',*,*,#20138,.T.);
#28669=ORIENTED_EDGE('',*,*,#20136,.T.);
#28670=ORIENTED_EDGE('',*,*,#20141,.T.);
#28671=ORIENTED_EDGE('',*,*,#20256,.T.);
#28672=ORIENTED_EDGE('',*,*,#20131,.T.);
#28673=ORIENTED_EDGE('',*,*,#20129,.T.);
#28674=ORIENTED_EDGE('',*,*,#20134,.T.);
#28675=ORIENTED_EDGE('',*,*,#20257,.T.);
#28676=ORIENTED_EDGE('',*,*,#20124,.T.);
#28677=ORIENTED_EDGE('',*,*,#20122,.T.);
#28678=ORIENTED_EDGE('',*,*,#20127,.T.);
#28679=ORIENTED_EDGE('',*,*,#20258,.T.);
#28680=ORIENTED_EDGE('',*,*,#20117,.T.);
#28681=ORIENTED_EDGE('',*,*,#20115,.T.);
#28682=ORIENTED_EDGE('',*,*,#20120,.T.);
#28683=ORIENTED_EDGE('',*,*,#20259,.T.);
#28684=ORIENTED_EDGE('',*,*,#20110,.T.);
#28685=ORIENTED_EDGE('',*,*,#20108,.T.);
#28686=ORIENTED_EDGE('',*,*,#20113,.T.);
#28687=ORIENTED_EDGE('',*,*,#20260,.T.);
#28688=ORIENTED_EDGE('',*,*,#20103,.T.);
#28689=ORIENTED_EDGE('',*,*,#20101,.T.);
#28690=ORIENTED_EDGE('',*,*,#20106,.T.);
#28691=ORIENTED_EDGE('',*,*,#20261,.T.);
#28692=ORIENTED_EDGE('',*,*,#20096,.T.);
#28693=ORIENTED_EDGE('',*,*,#20094,.T.);
#28694=ORIENTED_EDGE('',*,*,#20099,.T.);
#28695=ORIENTED_EDGE('',*,*,#20262,.T.);
#28696=ORIENTED_EDGE('',*,*,#20089,.T.);
#28697=ORIENTED_EDGE('',*,*,#20087,.T.);
#28698=ORIENTED_EDGE('',*,*,#20092,.T.);
#28699=ORIENTED_EDGE('',*,*,#20263,.T.);
#28700=ORIENTED_EDGE('',*,*,#20082,.T.);
#28701=ORIENTED_EDGE('',*,*,#20080,.T.);
#28702=ORIENTED_EDGE('',*,*,#20085,.T.);
#28703=ORIENTED_EDGE('',*,*,#20264,.T.);
#28704=ORIENTED_EDGE('',*,*,#20075,.T.);
#28705=ORIENTED_EDGE('',*,*,#20073,.T.);
#28706=ORIENTED_EDGE('',*,*,#20078,.T.);
#28707=ORIENTED_EDGE('',*,*,#20265,.T.);
#28708=ORIENTED_EDGE('',*,*,#20068,.T.);
#28709=ORIENTED_EDGE('',*,*,#20066,.T.);
#28710=ORIENTED_EDGE('',*,*,#20071,.T.);
#28711=ORIENTED_EDGE('',*,*,#20266,.T.);
#28712=ORIENTED_EDGE('',*,*,#20061,.T.);
#28713=ORIENTED_EDGE('',*,*,#20059,.T.);
#28714=ORIENTED_EDGE('',*,*,#20064,.T.);
#28715=ORIENTED_EDGE('',*,*,#20267,.T.);
#28716=ORIENTED_EDGE('',*,*,#20054,.T.);
#28717=ORIENTED_EDGE('',*,*,#20052,.T.);
#28718=ORIENTED_EDGE('',*,*,#20057,.T.);
#28719=ORIENTED_EDGE('',*,*,#20268,.T.);
#28720=ORIENTED_EDGE('',*,*,#20047,.T.);
#28721=ORIENTED_EDGE('',*,*,#20045,.T.);
#28722=ORIENTED_EDGE('',*,*,#20050,.T.);
#28723=ORIENTED_EDGE('',*,*,#20269,.T.);
#28724=ORIENTED_EDGE('',*,*,#20040,.T.);
#28725=ORIENTED_EDGE('',*,*,#20038,.T.);
#28726=ORIENTED_EDGE('',*,*,#20043,.T.);
#28727=ORIENTED_EDGE('',*,*,#20270,.T.);
#28728=ORIENTED_EDGE('',*,*,#20033,.T.);
#28729=ORIENTED_EDGE('',*,*,#20031,.T.);
#28730=ORIENTED_EDGE('',*,*,#20036,.T.);
#28731=ORIENTED_EDGE('',*,*,#20271,.T.);
#28732=ORIENTED_EDGE('',*,*,#20026,.T.);
#28733=ORIENTED_EDGE('',*,*,#20024,.T.);
#28734=ORIENTED_EDGE('',*,*,#20029,.T.);
#28735=ORIENTED_EDGE('',*,*,#20272,.T.);
#28736=ORIENTED_EDGE('',*,*,#20019,.T.);
#28737=ORIENTED_EDGE('',*,*,#20017,.T.);
#28738=ORIENTED_EDGE('',*,*,#20022,.T.);
#28739=ORIENTED_EDGE('',*,*,#20273,.T.);
#28740=ORIENTED_EDGE('',*,*,#20012,.T.);
#28741=ORIENTED_EDGE('',*,*,#20010,.T.);
#28742=ORIENTED_EDGE('',*,*,#20015,.T.);
#28743=ORIENTED_EDGE('',*,*,#20274,.T.);
#28744=ORIENTED_EDGE('',*,*,#20005,.T.);
#28745=ORIENTED_EDGE('',*,*,#20003,.T.);
#28746=ORIENTED_EDGE('',*,*,#20008,.T.);
#28747=ORIENTED_EDGE('',*,*,#20275,.T.);
#28748=ORIENTED_EDGE('',*,*,#19998,.T.);
#28749=ORIENTED_EDGE('',*,*,#19996,.T.);
#28750=ORIENTED_EDGE('',*,*,#20001,.T.);
#28751=ORIENTED_EDGE('',*,*,#20276,.T.);
#28752=ORIENTED_EDGE('',*,*,#19991,.T.);
#28753=ORIENTED_EDGE('',*,*,#19989,.T.);
#28754=ORIENTED_EDGE('',*,*,#19994,.T.);
#28755=ORIENTED_EDGE('',*,*,#20277,.T.);
#28756=ORIENTED_EDGE('',*,*,#19984,.T.);
#28757=ORIENTED_EDGE('',*,*,#19982,.T.);
#28758=ORIENTED_EDGE('',*,*,#19987,.T.);
#28759=ORIENTED_EDGE('',*,*,#20278,.T.);
#28760=ORIENTED_EDGE('',*,*,#19977,.T.);
#28761=ORIENTED_EDGE('',*,*,#19975,.T.);
#28762=ORIENTED_EDGE('',*,*,#19980,.T.);
#28763=ORIENTED_EDGE('',*,*,#20279,.T.);
#28764=ORIENTED_EDGE('',*,*,#19970,.T.);
#28765=ORIENTED_EDGE('',*,*,#19968,.T.);
#28766=ORIENTED_EDGE('',*,*,#19964,.T.);
#28767=ORIENTED_EDGE('',*,*,#19966,.T.);
#28768=ORIENTED_EDGE('',*,*,#19959,.T.);
#28769=ORIENTED_EDGE('',*,*,#19962,.T.);
#31663=PLANE('',#36752);
#31664=PLANE('',#36757);
#31665=PLANE('',#36918);
#31666=PLANE('',#36919);
#31667=PLANE('',#36922);
#31668=PLANE('',#37243);
#33155=ADVANCED_FACE('',(#5474),#908,.T.);
#33156=ADVANCED_FACE('',(#5475),#1589,.T.);
#33157=ADVANCED_FACE('',(#5476,#2134),#31663,.T.);
#33158=ADVANCED_FACE('',(#5477),#909,.F.);
#33159=ADVANCED_FACE('',(#5478,#2135),#31664,.F.);
#33160=ADVANCED_FACE('',(#5479),#31665,.F.);
#33161=ADVANCED_FACE('',(#5480),#31666,.F.);
#33162=ADVANCED_FACE('',(#5481),#1590,.F.);
#33163=ADVANCED_FACE('',(#5482),#31667,.F.);
#33164=ADVANCED_FACE('',(#5483),#1591,.T.);
#33165=ADVANCED_FACE('',(#5484),#1592,.T.);
#33166=ADVANCED_FACE('',(#5485),#1593,.T.);
#33167=ADVANCED_FACE('',(#5486),#1594,.T.);
#33168=ADVANCED_FACE('',(#5487),#1595,.T.);
#33169=ADVANCED_FACE('',(#5488),#1596,.T.);
#33170=ADVANCED_FACE('',(#5489),#1597,.T.);
#33171=ADVANCED_FACE('',(#5490),#1598,.T.);
#33172=ADVANCED_FACE('',(#5491),#1599,.T.);
#33173=ADVANCED_FACE('',(#5492),#1600,.T.);
#33174=ADVANCED_FACE('',(#5493),#1601,.T.);
#33175=ADVANCED_FACE('',(#5494),#1602,.T.);
#33176=ADVANCED_FACE('',(#5495),#1603,.T.);
#33177=ADVANCED_FACE('',(#5496),#1604,.T.);
#33178=ADVANCED_FACE('',(#5497),#1605,.T.);
#33179=ADVANCED_FACE('',(#5498),#1606,.T.);
#33180=ADVANCED_FACE('',(#5499),#1607,.T.);
#33181=ADVANCED_FACE('',(#5500),#1608,.T.);
#33182=ADVANCED_FACE('',(#5501),#1609,.T.);
#33183=ADVANCED_FACE('',(#5502),#1610,.T.);
#33184=ADVANCED_FACE('',(#5503),#1611,.T.);
#33185=ADVANCED_FACE('',(#5504),#1612,.T.);
#33186=ADVANCED_FACE('',(#5505),#1613,.T.);
#33187=ADVANCED_FACE('',(#5506),#1614,.T.);
#33188=ADVANCED_FACE('',(#5507),#1615,.T.);
#33189=ADVANCED_FACE('',(#5508),#1616,.T.);
#33190=ADVANCED_FACE('',(#5509),#1617,.T.);
#33191=ADVANCED_FACE('',(#5510),#1618,.T.);
#33192=ADVANCED_FACE('',(#5511),#1619,.T.);
#33193=ADVANCED_FACE('',(#5512),#1620,.T.);
#33194=ADVANCED_FACE('',(#5513),#1621,.T.);
#33195=ADVANCED_FACE('',(#5514),#1622,.T.);
#33196=ADVANCED_FACE('',(#5515),#1623,.T.);
#33197=ADVANCED_FACE('',(#5516),#1624,.T.);
#33198=ADVANCED_FACE('',(#5517),#1625,.T.);
#33199=ADVANCED_FACE('',(#5518),#1626,.T.);
#33200=ADVANCED_FACE('',(#5519),#1627,.T.);
#33201=ADVANCED_FACE('',(#5520),#1628,.T.);
#33202=ADVANCED_FACE('',(#5521),#1629,.T.);
#33203=ADVANCED_FACE('',(#5522),#1630,.T.);
#33204=ADVANCED_FACE('',(#5523),#1631,.T.);
#33205=ADVANCED_FACE('',(#5524),#1632,.T.);
#33206=ADVANCED_FACE('',(#5525),#1633,.T.);
#33207=ADVANCED_FACE('',(#5526),#1634,.T.);
#33208=ADVANCED_FACE('',(#5527),#1635,.T.);
#33209=ADVANCED_FACE('',(#5528),#1636,.T.);
#33210=ADVANCED_FACE('',(#5529),#1637,.T.);
#33211=ADVANCED_FACE('',(#5530),#1638,.T.);
#33212=ADVANCED_FACE('',(#5531),#1639,.T.);
#33213=ADVANCED_FACE('',(#5532),#1640,.T.);
#33214=ADVANCED_FACE('',(#5533),#1641,.T.);
#33215=ADVANCED_FACE('',(#5534),#1642,.T.);
#33216=ADVANCED_FACE('',(#5535),#1643,.T.);
#33217=ADVANCED_FACE('',(#5536),#1644,.T.);
#33218=ADVANCED_FACE('',(#5537),#1645,.T.);
#33219=ADVANCED_FACE('',(#5538),#1646,.T.);
#33220=ADVANCED_FACE('',(#5539),#1647,.T.);
#33221=ADVANCED_FACE('',(#5540),#1648,.T.);
#33222=ADVANCED_FACE('',(#5541),#1649,.T.);
#33223=ADVANCED_FACE('',(#5542),#1650,.T.);
#33224=ADVANCED_FACE('',(#5543),#1651,.T.);
#33225=ADVANCED_FACE('',(#5544),#1652,.T.);
#33226=ADVANCED_FACE('',(#5545),#1653,.T.);
#33227=ADVANCED_FACE('',(#5546),#1654,.T.);
#33228=ADVANCED_FACE('',(#5547),#1655,.T.);
#33229=ADVANCED_FACE('',(#5548),#1656,.T.);
#33230=ADVANCED_FACE('',(#5549),#1657,.T.);
#33231=ADVANCED_FACE('',(#5550),#1658,.T.);
#33232=ADVANCED_FACE('',(#5551),#1659,.T.);
#33233=ADVANCED_FACE('',(#5552),#1660,.T.);
#33234=ADVANCED_FACE('',(#5553),#1661,.T.);
#33235=ADVANCED_FACE('',(#5554),#1662,.T.);
#33236=ADVANCED_FACE('',(#5555),#1663,.T.);
#33237=ADVANCED_FACE('',(#5556),#1664,.T.);
#33238=ADVANCED_FACE('',(#5557),#1665,.T.);
#33239=ADVANCED_FACE('',(#5558),#1666,.T.);
#33240=ADVANCED_FACE('',(#5559),#1667,.T.);
#33241=ADVANCED_FACE('',(#5560),#1668,.T.);
#33242=ADVANCED_FACE('',(#5561),#1669,.T.);
#33243=ADVANCED_FACE('',(#5562),#1670,.T.);
#33244=ADVANCED_FACE('',(#5563),#1671,.T.);
#33245=ADVANCED_FACE('',(#5564),#1672,.T.);
#33246=ADVANCED_FACE('',(#5565),#1673,.T.);
#33247=ADVANCED_FACE('',(#5566),#1674,.T.);
#33248=ADVANCED_FACE('',(#5567),#1675,.T.);
#33249=ADVANCED_FACE('',(#5568),#1676,.T.);
#33250=ADVANCED_FACE('',(#5569),#1677,.T.);
#33251=ADVANCED_FACE('',(#5570),#1678,.T.);
#33252=ADVANCED_FACE('',(#5571),#1679,.T.);
#33253=ADVANCED_FACE('',(#5572),#1680,.T.);
#33254=ADVANCED_FACE('',(#5573),#1681,.T.);
#33255=ADVANCED_FACE('',(#5574),#1682,.T.);
#33256=ADVANCED_FACE('',(#5575),#1683,.T.);
#33257=ADVANCED_FACE('',(#5576),#1684,.T.);
#33258=ADVANCED_FACE('',(#5577),#1685,.T.);
#33259=ADVANCED_FACE('',(#5578),#1686,.T.);
#33260=ADVANCED_FACE('',(#5579),#1687,.T.);
#33261=ADVANCED_FACE('',(#5580),#1688,.T.);
#33262=ADVANCED_FACE('',(#5581),#1689,.T.);
#33263=ADVANCED_FACE('',(#5582),#1690,.T.);
#33264=ADVANCED_FACE('',(#5583),#1691,.T.);
#33265=ADVANCED_FACE('',(#5584),#1692,.T.);
#33266=ADVANCED_FACE('',(#5585),#1693,.T.);
#33267=ADVANCED_FACE('',(#5586),#1694,.T.);
#33268=ADVANCED_FACE('',(#5587),#1695,.T.);
#33269=ADVANCED_FACE('',(#5588),#1696,.T.);
#33270=ADVANCED_FACE('',(#5589),#1697,.T.);
#33271=ADVANCED_FACE('',(#5590),#1698,.T.);
#33272=ADVANCED_FACE('',(#5591),#1699,.T.);
#33273=ADVANCED_FACE('',(#5592),#1700,.T.);
#33274=ADVANCED_FACE('',(#5593),#1701,.T.);
#33275=ADVANCED_FACE('',(#5594),#1702,.T.);
#33276=ADVANCED_FACE('',(#5595),#1703,.T.);
#33277=ADVANCED_FACE('',(#5596),#1704,.T.);
#33278=ADVANCED_FACE('',(#5597),#1705,.T.);
#33279=ADVANCED_FACE('',(#5598),#1706,.T.);
#33280=ADVANCED_FACE('',(#5599),#1707,.T.);
#33281=ADVANCED_FACE('',(#5600),#1708,.T.);
#33282=ADVANCED_FACE('',(#5601),#1709,.T.);
#33283=ADVANCED_FACE('',(#5602),#1710,.T.);
#33284=ADVANCED_FACE('',(#5603),#1711,.T.);
#33285=ADVANCED_FACE('',(#5604),#1712,.T.);
#33286=ADVANCED_FACE('',(#5605),#1713,.T.);
#33287=ADVANCED_FACE('',(#5606),#1714,.T.);
#33288=ADVANCED_FACE('',(#5607),#1715,.T.);
#33289=ADVANCED_FACE('',(#5608),#1716,.T.);
#33290=ADVANCED_FACE('',(#5609),#1717,.T.);
#33291=ADVANCED_FACE('',(#5610),#1718,.T.);
#33292=ADVANCED_FACE('',(#5611),#1719,.T.);
#33293=ADVANCED_FACE('',(#5612),#1720,.T.);
#33294=ADVANCED_FACE('',(#5613),#1721,.T.);
#33295=ADVANCED_FACE('',(#5614),#1722,.T.);
#33296=ADVANCED_FACE('',(#5615),#1723,.T.);
#33297=ADVANCED_FACE('',(#5616),#1724,.T.);
#33298=ADVANCED_FACE('',(#5617),#1725,.T.);
#33299=ADVANCED_FACE('',(#5618),#1726,.T.);
#33300=ADVANCED_FACE('',(#5619),#1727,.T.);
#33301=ADVANCED_FACE('',(#5620),#1728,.T.);
#33302=ADVANCED_FACE('',(#5621),#1729,.T.);
#33303=ADVANCED_FACE('',(#5622),#1730,.T.);
#33304=ADVANCED_FACE('',(#5623),#1731,.T.);
#33305=ADVANCED_FACE('',(#5624),#1732,.T.);
#33306=ADVANCED_FACE('',(#5625),#1733,.T.);
#33307=ADVANCED_FACE('',(#5626),#1734,.T.);
#33308=ADVANCED_FACE('',(#5627),#1735,.T.);
#33309=ADVANCED_FACE('',(#5628),#1736,.T.);
#33310=ADVANCED_FACE('',(#5629),#1737,.T.);
#33311=ADVANCED_FACE('',(#5630),#1738,.T.);
#33312=ADVANCED_FACE('',(#5631),#1739,.T.);
#33313=ADVANCED_FACE('',(#5632),#1740,.T.);
#33314=ADVANCED_FACE('',(#5633),#1741,.T.);
#33315=ADVANCED_FACE('',(#5634),#1742,.T.);
#33316=ADVANCED_FACE('',(#5635),#1743,.T.);
#33317=ADVANCED_FACE('',(#5636),#1744,.T.);
#33318=ADVANCED_FACE('',(#5637),#1745,.T.);
#33319=ADVANCED_FACE('',(#5638),#1746,.T.);
#33320=ADVANCED_FACE('',(#5639),#1747,.T.);
#33321=ADVANCED_FACE('',(#5640),#1748,.T.);
#33322=ADVANCED_FACE('',(#5641),#1749,.T.);
#33323=ADVANCED_FACE('',(#5642),#1750,.T.);
#33324=ADVANCED_FACE('',(#5643,#2136),#31668,.T.);
#33827=CLOSED_SHELL('',(#33155,#33156,#33157,#33158,#33159,#33160,#33161,
#33162,#33163,#33164,#33165,#33166,#33167,#33168,#33169,#33170,#33171,#33172,
#33173,#33174,#33175,#33176,#33177,#33178,#33179,#33180,#33181,#33182,#33183,
#33184,#33185,#33186,#33187,#33188,#33189,#33190,#33191,#33192,#33193,#33194,
#33195,#33196,#33197,#33198,#33199,#33200,#33201,#33202,#33203,#33204,#33205,
#33206,#33207,#33208,#33209,#33210,#33211,#33212,#33213,#33214,#33215,#33216,
#33217,#33218,#33219,#33220,#33221,#33222,#33223,#33224,#33225,#33226,#33227,
#33228,#33229,#33230,#33231,#33232,#33233,#33234,#33235,#33236,#33237,#33238,
#33239,#33240,#33241,#33242,#33243,#33244,#33245,#33246,#33247,#33248,#33249,
#33250,#33251,#33252,#33253,#33254,#33255,#33256,#33257,#33258,#33259,#33260,
#33261,#33262,#33263,#33264,#33265,#33266,#33267,#33268,#33269,#33270,#33271,
#33272,#33273,#33274,#33275,#33276,#33277,#33278,#33279,#33280,#33281,#33282,
#33283,#33284,#33285,#33286,#33287,#33288,#33289,#33290,#33291,#33292,#33293,
#33294,#33295,#33296,#33297,#33298,#33299,#33300,#33301,#33302,#33303,#33304,
#33305,#33306,#33307,#33308,#33309,#33310,#33311,#33312,#33313,#33314,#33315,
#33316,#33317,#33318,#33319,#33320,#33321,#33322,#33323,#33324));
#36744=AXIS2_PLACEMENT_3D('',#57600,#45113,#45114);
#36745=AXIS2_PLACEMENT_3D('',#57601,#45115,#45116);
#36746=AXIS2_PLACEMENT_3D('',#57603,#45117,#45118);
#36747=AXIS2_PLACEMENT_3D('',#57605,#45119,#45120);
#36748=AXIS2_PLACEMENT_3D('',#57607,#45121,#45122);
#36749=AXIS2_PLACEMENT_3D('',#57608,#45123,#45124);
#36750=AXIS2_PLACEMENT_3D('',#57609,#45125,#45126);
#36751=AXIS2_PLACEMENT_3D('',#57612,#45128,#45129);
#36752=AXIS2_PLACEMENT_3D('',#57613,#45130,#45131);
#36753=AXIS2_PLACEMENT_3D('',#57621,#45135,#45136);
#36754=AXIS2_PLACEMENT_3D('',#57622,#45137,#45138);
#36755=AXIS2_PLACEMENT_3D('',#57624,#45139,#45140);
#36756=AXIS2_PLACEMENT_3D('',#57625,#45141,#45142);
#36757=AXIS2_PLACEMENT_3D('',#57626,#45143,#45144);
#36758=AXIS2_PLACEMENT_3D('',#57629,#45145,#45146);
#36759=AXIS2_PLACEMENT_3D('',#57631,#45147,#45148);
#36760=AXIS2_PLACEMENT_3D('',#57633,#45149,#45150);
#36761=AXIS2_PLACEMENT_3D('',#57635,#45151,#45152);
#36762=AXIS2_PLACEMENT_3D('',#57637,#45153,#45154);
#36763=AXIS2_PLACEMENT_3D('',#57639,#45155,#45156);
#36764=AXIS2_PLACEMENT_3D('',#57641,#45157,#45158);
#36765=AXIS2_PLACEMENT_3D('',#57643,#45159,#45160);
#36766=AXIS2_PLACEMENT_3D('',#57645,#45161,#45162);
#36767=AXIS2_PLACEMENT_3D('',#57647,#45163,#45164);
#36768=AXIS2_PLACEMENT_3D('',#57649,#45165,#45166);
#36769=AXIS2_PLACEMENT_3D('',#57651,#45167,#45168);
#36770=AXIS2_PLACEMENT_3D('',#57653,#45169,#45170);
#36771=AXIS2_PLACEMENT_3D('',#57655,#45171,#45172);
#36772=AXIS2_PLACEMENT_3D('',#57657,#45173,#45174);
#36773=AXIS2_PLACEMENT_3D('',#57659,#45175,#45176);
#36774=AXIS2_PLACEMENT_3D('',#57661,#45177,#45178);
#36775=AXIS2_PLACEMENT_3D('',#57663,#45179,#45180);
#36776=AXIS2_PLACEMENT_3D('',#57665,#45181,#45182);
#36777=AXIS2_PLACEMENT_3D('',#57667,#45183,#45184);
#36778=AXIS2_PLACEMENT_3D('',#57669,#45185,#45186);
#36779=AXIS2_PLACEMENT_3D('',#57671,#45187,#45188);
#36780=AXIS2_PLACEMENT_3D('',#57673,#45189,#45190);
#36781=AXIS2_PLACEMENT_3D('',#57675,#45191,#45192);
#36782=AXIS2_PLACEMENT_3D('',#57677,#45193,#45194);
#36783=AXIS2_PLACEMENT_3D('',#57679,#45195,#45196);
#36784=AXIS2_PLACEMENT_3D('',#57681,#45197,#45198);
#36785=AXIS2_PLACEMENT_3D('',#57683,#45199,#45200);
#36786=AXIS2_PLACEMENT_3D('',#57685,#45201,#45202);
#36787=AXIS2_PLACEMENT_3D('',#57687,#45203,#45204);
#36788=AXIS2_PLACEMENT_3D('',#57689,#45205,#45206);
#36789=AXIS2_PLACEMENT_3D('',#57691,#45207,#45208);
#36790=AXIS2_PLACEMENT_3D('',#57693,#45209,#45210);
#36791=AXIS2_PLACEMENT_3D('',#57695,#45211,#45212);
#36792=AXIS2_PLACEMENT_3D('',#57697,#45213,#45214);
#36793=AXIS2_PLACEMENT_3D('',#57699,#45215,#45216);
#36794=AXIS2_PLACEMENT_3D('',#57701,#45217,#45218);
#36795=AXIS2_PLACEMENT_3D('',#57703,#45219,#45220);
#36796=AXIS2_PLACEMENT_3D('',#57705,#45221,#45222);
#36797=AXIS2_PLACEMENT_3D('',#57707,#45223,#45224);
#36798=AXIS2_PLACEMENT_3D('',#57709,#45225,#45226);
#36799=AXIS2_PLACEMENT_3D('',#57711,#45227,#45228);
#36800=AXIS2_PLACEMENT_3D('',#57713,#45229,#45230);
#36801=AXIS2_PLACEMENT_3D('',#57715,#45231,#45232);
#36802=AXIS2_PLACEMENT_3D('',#57717,#45233,#45234);
#36803=AXIS2_PLACEMENT_3D('',#57719,#45235,#45236);
#36804=AXIS2_PLACEMENT_3D('',#57721,#45237,#45238);
#36805=AXIS2_PLACEMENT_3D('',#57723,#45239,#45240);
#36806=AXIS2_PLACEMENT_3D('',#57725,#45241,#45242);
#36807=AXIS2_PLACEMENT_3D('',#57727,#45243,#45244);
#36808=AXIS2_PLACEMENT_3D('',#57729,#45245,#45246);
#36809=AXIS2_PLACEMENT_3D('',#57731,#45247,#45248);
#36810=AXIS2_PLACEMENT_3D('',#57733,#45249,#45250);
#36811=AXIS2_PLACEMENT_3D('',#57735,#45251,#45252);
#36812=AXIS2_PLACEMENT_3D('',#57737,#45253,#45254);
#36813=AXIS2_PLACEMENT_3D('',#57739,#45255,#45256);
#36814=AXIS2_PLACEMENT_3D('',#57741,#45257,#45258);
#36815=AXIS2_PLACEMENT_3D('',#57743,#45259,#45260);
#36816=AXIS2_PLACEMENT_3D('',#57745,#45261,#45262);
#36817=AXIS2_PLACEMENT_3D('',#57747,#45263,#45264);
#36818=AXIS2_PLACEMENT_3D('',#57749,#45265,#45266);
#36819=AXIS2_PLACEMENT_3D('',#57751,#45267,#45268);
#36820=AXIS2_PLACEMENT_3D('',#57753,#45269,#45270);
#36821=AXIS2_PLACEMENT_3D('',#57755,#45271,#45272);
#36822=AXIS2_PLACEMENT_3D('',#57757,#45273,#45274);
#36823=AXIS2_PLACEMENT_3D('',#57759,#45275,#45276);
#36824=AXIS2_PLACEMENT_3D('',#57761,#45277,#45278);
#36825=AXIS2_PLACEMENT_3D('',#57763,#45279,#45280);
#36826=AXIS2_PLACEMENT_3D('',#57765,#45281,#45282);
#36827=AXIS2_PLACEMENT_3D('',#57767,#45283,#45284);
#36828=AXIS2_PLACEMENT_3D('',#57769,#45285,#45286);
#36829=AXIS2_PLACEMENT_3D('',#57771,#45287,#45288);
#36830=AXIS2_PLACEMENT_3D('',#57773,#45289,#45290);
#36831=AXIS2_PLACEMENT_3D('',#57775,#45291,#45292);
#36832=AXIS2_PLACEMENT_3D('',#57777,#45293,#45294);
#36833=AXIS2_PLACEMENT_3D('',#57779,#45295,#45296);
#36834=AXIS2_PLACEMENT_3D('',#57781,#45297,#45298);
#36835=AXIS2_PLACEMENT_3D('',#57783,#45299,#45300);
#36836=AXIS2_PLACEMENT_3D('',#57785,#45301,#45302);
#36837=AXIS2_PLACEMENT_3D('',#57787,#45303,#45304);
#36838=AXIS2_PLACEMENT_3D('',#57789,#45305,#45306);
#36839=AXIS2_PLACEMENT_3D('',#57791,#45307,#45308);
#36840=AXIS2_PLACEMENT_3D('',#57793,#45309,#45310);
#36841=AXIS2_PLACEMENT_3D('',#57795,#45311,#45312);
#36842=AXIS2_PLACEMENT_3D('',#57797,#45313,#45314);
#36843=AXIS2_PLACEMENT_3D('',#57799,#45315,#45316);
#36844=AXIS2_PLACEMENT_3D('',#57801,#45317,#45318);
#36845=AXIS2_PLACEMENT_3D('',#57803,#45319,#45320);
#36846=AXIS2_PLACEMENT_3D('',#57805,#45321,#45322);
#36847=AXIS2_PLACEMENT_3D('',#57807,#45323,#45324);
#36848=AXIS2_PLACEMENT_3D('',#57809,#45325,#45326);
#36849=AXIS2_PLACEMENT_3D('',#57811,#45327,#45328);
#36850=AXIS2_PLACEMENT_3D('',#57813,#45329,#45330);
#36851=AXIS2_PLACEMENT_3D('',#57815,#45331,#45332);
#36852=AXIS2_PLACEMENT_3D('',#57817,#45333,#45334);
#36853=AXIS2_PLACEMENT_3D('',#57819,#45335,#45336);
#36854=AXIS2_PLACEMENT_3D('',#57821,#45337,#45338);
#36855=AXIS2_PLACEMENT_3D('',#57823,#45339,#45340);
#36856=AXIS2_PLACEMENT_3D('',#57825,#45341,#45342);
#36857=AXIS2_PLACEMENT_3D('',#57827,#45343,#45344);
#36858=AXIS2_PLACEMENT_3D('',#57829,#45345,#45346);
#36859=AXIS2_PLACEMENT_3D('',#57831,#45347,#45348);
#36860=AXIS2_PLACEMENT_3D('',#57833,#45349,#45350);
#36861=AXIS2_PLACEMENT_3D('',#57835,#45351,#45352);
#36862=AXIS2_PLACEMENT_3D('',#57837,#45353,#45354);
#36863=AXIS2_PLACEMENT_3D('',#57839,#45355,#45356);
#36864=AXIS2_PLACEMENT_3D('',#57841,#45357,#45358);
#36865=AXIS2_PLACEMENT_3D('',#57843,#45359,#45360);
#36866=AXIS2_PLACEMENT_3D('',#57845,#45361,#45362);
#36867=AXIS2_PLACEMENT_3D('',#57847,#45363,#45364);
#36868=AXIS2_PLACEMENT_3D('',#57849,#45365,#45366);
#36869=AXIS2_PLACEMENT_3D('',#57851,#45367,#45368);
#36870=AXIS2_PLACEMENT_3D('',#57853,#45369,#45370);
#36871=AXIS2_PLACEMENT_3D('',#57855,#45371,#45372);
#36872=AXIS2_PLACEMENT_3D('',#57857,#45373,#45374);
#36873=AXIS2_PLACEMENT_3D('',#57859,#45375,#45376);
#36874=AXIS2_PLACEMENT_3D('',#57861,#45377,#45378);
#36875=AXIS2_PLACEMENT_3D('',#57863,#45379,#45380);
#36876=AXIS2_PLACEMENT_3D('',#57865,#45381,#45382);
#36877=AXIS2_PLACEMENT_3D('',#57867,#45383,#45384);
#36878=AXIS2_PLACEMENT_3D('',#57869,#45385,#45386);
#36879=AXIS2_PLACEMENT_3D('',#57871,#45387,#45388);
#36880=AXIS2_PLACEMENT_3D('',#57873,#45389,#45390);
#36881=AXIS2_PLACEMENT_3D('',#57875,#45391,#45392);
#36882=AXIS2_PLACEMENT_3D('',#57877,#45393,#45394);
#36883=AXIS2_PLACEMENT_3D('',#57879,#45395,#45396);
#36884=AXIS2_PLACEMENT_3D('',#57881,#45397,#45398);
#36885=AXIS2_PLACEMENT_3D('',#57883,#45399,#45400);
#36886=AXIS2_PLACEMENT_3D('',#57885,#45401,#45402);
#36887=AXIS2_PLACEMENT_3D('',#57887,#45403,#45404);
#36888=AXIS2_PLACEMENT_3D('',#57889,#45405,#45406);
#36889=AXIS2_PLACEMENT_3D('',#57891,#45407,#45408);
#36890=AXIS2_PLACEMENT_3D('',#57893,#45409,#45410);
#36891=AXIS2_PLACEMENT_3D('',#57895,#45411,#45412);
#36892=AXIS2_PLACEMENT_3D('',#57897,#45413,#45414);
#36893=AXIS2_PLACEMENT_3D('',#57899,#45415,#45416);
#36894=AXIS2_PLACEMENT_3D('',#57901,#45417,#45418);
#36895=AXIS2_PLACEMENT_3D('',#57903,#45419,#45420);
#36896=AXIS2_PLACEMENT_3D('',#57905,#45421,#45422);
#36897=AXIS2_PLACEMENT_3D('',#57907,#45423,#45424);
#36898=AXIS2_PLACEMENT_3D('',#57909,#45425,#45426);
#36899=AXIS2_PLACEMENT_3D('',#57911,#45427,#45428);
#36900=AXIS2_PLACEMENT_3D('',#57913,#45429,#45430);
#36901=AXIS2_PLACEMENT_3D('',#57915,#45431,#45432);
#36902=AXIS2_PLACEMENT_3D('',#57917,#45433,#45434);
#36903=AXIS2_PLACEMENT_3D('',#57919,#45435,#45436);
#36904=AXIS2_PLACEMENT_3D('',#57921,#45437,#45438);
#36905=AXIS2_PLACEMENT_3D('',#57923,#45439,#45440);
#36906=AXIS2_PLACEMENT_3D('',#57925,#45441,#45442);
#36907=AXIS2_PLACEMENT_3D('',#57927,#45443,#45444);
#36908=AXIS2_PLACEMENT_3D('',#57929,#45445,#45446);
#36909=AXIS2_PLACEMENT_3D('',#57931,#45447,#45448);
#36910=AXIS2_PLACEMENT_3D('',#57933,#45449,#45450);
#36911=AXIS2_PLACEMENT_3D('',#57935,#45451,#45452);
#36912=AXIS2_PLACEMENT_3D('',#57937,#45453,#45454);
#36913=AXIS2_PLACEMENT_3D('',#57939,#45455,#45456);
#36914=AXIS2_PLACEMENT_3D('',#57941,#45457,#45458);
#36915=AXIS2_PLACEMENT_3D('',#57943,#45459,#45460);
#36916=AXIS2_PLACEMENT_3D('',#57945,#45461,#45462);
#36917=AXIS2_PLACEMENT_3D('',#57946,#45463,#45464);
#36918=AXIS2_PLACEMENT_3D('',#57947,#45465,#45466);
#36919=AXIS2_PLACEMENT_3D('',#57953,#45470,#45471);
#36920=AXIS2_PLACEMENT_3D('',#57957,#45474,#45475);
#36921=AXIS2_PLACEMENT_3D('',#57959,#45476,#45477);
#36922=AXIS2_PLACEMENT_3D('',#57961,#45479,#45480);
#36923=AXIS2_PLACEMENT_3D('',#57963,#45482,#45483);
#36924=AXIS2_PLACEMENT_3D('',#57967,#45485,#45486);
#36925=AXIS2_PLACEMENT_3D('',#57969,#45488,#45489);
#36926=AXIS2_PLACEMENT_3D('',#57971,#45490,#45491);
#36927=AXIS2_PLACEMENT_3D('',#57973,#45493,#45494);
#36928=AXIS2_PLACEMENT_3D('',#57976,#45496,#45497);
#36929=AXIS2_PLACEMENT_3D('',#57977,#45498,#45499);
#36930=AXIS2_PLACEMENT_3D('',#57981,#45501,#45502);
#36931=AXIS2_PLACEMENT_3D('',#57983,#45504,#45505);
#36932=AXIS2_PLACEMENT_3D('',#57985,#45506,#45507);
#36933=AXIS2_PLACEMENT_3D('',#57987,#45509,#45510);
#36934=AXIS2_PLACEMENT_3D('',#57990,#45512,#45513);
#36935=AXIS2_PLACEMENT_3D('',#57991,#45514,#45515);
#36936=AXIS2_PLACEMENT_3D('',#57995,#45517,#45518);
#36937=AXIS2_PLACEMENT_3D('',#57997,#45520,#45521);
#36938=AXIS2_PLACEMENT_3D('',#57999,#45522,#45523);
#36939=AXIS2_PLACEMENT_3D('',#58001,#45525,#45526);
#36940=AXIS2_PLACEMENT_3D('',#58004,#45528,#45529);
#36941=AXIS2_PLACEMENT_3D('',#58005,#45530,#45531);
#36942=AXIS2_PLACEMENT_3D('',#58009,#45533,#45534);
#36943=AXIS2_PLACEMENT_3D('',#58011,#45536,#45537);
#36944=AXIS2_PLACEMENT_3D('',#58013,#45538,#45539);
#36945=AXIS2_PLACEMENT_3D('',#58015,#45541,#45542);
#36946=AXIS2_PLACEMENT_3D('',#58018,#45544,#45545);
#36947=AXIS2_PLACEMENT_3D('',#58019,#45546,#45547);
#36948=AXIS2_PLACEMENT_3D('',#58023,#45549,#45550);
#36949=AXIS2_PLACEMENT_3D('',#58025,#45552,#45553);
#36950=AXIS2_PLACEMENT_3D('',#58027,#45554,#45555);
#36951=AXIS2_PLACEMENT_3D('',#58029,#45557,#45558);
#36952=AXIS2_PLACEMENT_3D('',#58032,#45560,#45561);
#36953=AXIS2_PLACEMENT_3D('',#58033,#45562,#45563);
#36954=AXIS2_PLACEMENT_3D('',#58037,#45565,#45566);
#36955=AXIS2_PLACEMENT_3D('',#58039,#45568,#45569);
#36956=AXIS2_PLACEMENT_3D('',#58041,#45570,#45571);
#36957=AXIS2_PLACEMENT_3D('',#58043,#45573,#45574);
#36958=AXIS2_PLACEMENT_3D('',#58046,#45576,#45577);
#36959=AXIS2_PLACEMENT_3D('',#58047,#45578,#45579);
#36960=AXIS2_PLACEMENT_3D('',#58051,#45581,#45582);
#36961=AXIS2_PLACEMENT_3D('',#58053,#45584,#45585);
#36962=AXIS2_PLACEMENT_3D('',#58055,#45586,#45587);
#36963=AXIS2_PLACEMENT_3D('',#58057,#45589,#45590);
#36964=AXIS2_PLACEMENT_3D('',#58060,#45592,#45593);
#36965=AXIS2_PLACEMENT_3D('',#58061,#45594,#45595);
#36966=AXIS2_PLACEMENT_3D('',#58065,#45597,#45598);
#36967=AXIS2_PLACEMENT_3D('',#58067,#45600,#45601);
#36968=AXIS2_PLACEMENT_3D('',#58069,#45602,#45603);
#36969=AXIS2_PLACEMENT_3D('',#58071,#45605,#45606);
#36970=AXIS2_PLACEMENT_3D('',#58074,#45608,#45609);
#36971=AXIS2_PLACEMENT_3D('',#58075,#45610,#45611);
#36972=AXIS2_PLACEMENT_3D('',#58079,#45613,#45614);
#36973=AXIS2_PLACEMENT_3D('',#58081,#45616,#45617);
#36974=AXIS2_PLACEMENT_3D('',#58083,#45618,#45619);
#36975=AXIS2_PLACEMENT_3D('',#58085,#45621,#45622);
#36976=AXIS2_PLACEMENT_3D('',#58088,#45624,#45625);
#36977=AXIS2_PLACEMENT_3D('',#58089,#45626,#45627);
#36978=AXIS2_PLACEMENT_3D('',#58093,#45629,#45630);
#36979=AXIS2_PLACEMENT_3D('',#58095,#45632,#45633);
#36980=AXIS2_PLACEMENT_3D('',#58097,#45634,#45635);
#36981=AXIS2_PLACEMENT_3D('',#58099,#45637,#45638);
#36982=AXIS2_PLACEMENT_3D('',#58102,#45640,#45641);
#36983=AXIS2_PLACEMENT_3D('',#58103,#45642,#45643);
#36984=AXIS2_PLACEMENT_3D('',#58107,#45645,#45646);
#36985=AXIS2_PLACEMENT_3D('',#58109,#45648,#45649);
#36986=AXIS2_PLACEMENT_3D('',#58111,#45650,#45651);
#36987=AXIS2_PLACEMENT_3D('',#58113,#45653,#45654);
#36988=AXIS2_PLACEMENT_3D('',#58116,#45656,#45657);
#36989=AXIS2_PLACEMENT_3D('',#58117,#45658,#45659);
#36990=AXIS2_PLACEMENT_3D('',#58121,#45661,#45662);
#36991=AXIS2_PLACEMENT_3D('',#58123,#45664,#45665);
#36992=AXIS2_PLACEMENT_3D('',#58125,#45666,#45667);
#36993=AXIS2_PLACEMENT_3D('',#58127,#45669,#45670);
#36994=AXIS2_PLACEMENT_3D('',#58130,#45672,#45673);
#36995=AXIS2_PLACEMENT_3D('',#58131,#45674,#45675);
#36996=AXIS2_PLACEMENT_3D('',#58135,#45677,#45678);
#36997=AXIS2_PLACEMENT_3D('',#58137,#45680,#45681);
#36998=AXIS2_PLACEMENT_3D('',#58139,#45682,#45683);
#36999=AXIS2_PLACEMENT_3D('',#58141,#45685,#45686);
#37000=AXIS2_PLACEMENT_3D('',#58144,#45688,#45689);
#37001=AXIS2_PLACEMENT_3D('',#58145,#45690,#45691);
#37002=AXIS2_PLACEMENT_3D('',#58149,#45693,#45694);
#37003=AXIS2_PLACEMENT_3D('',#58151,#45696,#45697);
#37004=AXIS2_PLACEMENT_3D('',#58153,#45698,#45699);
#37005=AXIS2_PLACEMENT_3D('',#58155,#45701,#45702);
#37006=AXIS2_PLACEMENT_3D('',#58158,#45704,#45705);
#37007=AXIS2_PLACEMENT_3D('',#58159,#45706,#45707);
#37008=AXIS2_PLACEMENT_3D('',#58163,#45709,#45710);
#37009=AXIS2_PLACEMENT_3D('',#58165,#45712,#45713);
#37010=AXIS2_PLACEMENT_3D('',#58167,#45714,#45715);
#37011=AXIS2_PLACEMENT_3D('',#58169,#45717,#45718);
#37012=AXIS2_PLACEMENT_3D('',#58172,#45720,#45721);
#37013=AXIS2_PLACEMENT_3D('',#58173,#45722,#45723);
#37014=AXIS2_PLACEMENT_3D('',#58177,#45725,#45726);
#37015=AXIS2_PLACEMENT_3D('',#58179,#45728,#45729);
#37016=AXIS2_PLACEMENT_3D('',#58181,#45730,#45731);
#37017=AXIS2_PLACEMENT_3D('',#58183,#45733,#45734);
#37018=AXIS2_PLACEMENT_3D('',#58186,#45736,#45737);
#37019=AXIS2_PLACEMENT_3D('',#58187,#45738,#45739);
#37020=AXIS2_PLACEMENT_3D('',#58191,#45741,#45742);
#37021=AXIS2_PLACEMENT_3D('',#58193,#45744,#45745);
#37022=AXIS2_PLACEMENT_3D('',#58195,#45746,#45747);
#37023=AXIS2_PLACEMENT_3D('',#58197,#45749,#45750);
#37024=AXIS2_PLACEMENT_3D('',#58200,#45752,#45753);
#37025=AXIS2_PLACEMENT_3D('',#58201,#45754,#45755);
#37026=AXIS2_PLACEMENT_3D('',#58205,#45757,#45758);
#37027=AXIS2_PLACEMENT_3D('',#58207,#45760,#45761);
#37028=AXIS2_PLACEMENT_3D('',#58209,#45762,#45763);
#37029=AXIS2_PLACEMENT_3D('',#58211,#45765,#45766);
#37030=AXIS2_PLACEMENT_3D('',#58214,#45768,#45769);
#37031=AXIS2_PLACEMENT_3D('',#58215,#45770,#45771);
#37032=AXIS2_PLACEMENT_3D('',#58219,#45773,#45774);
#37033=AXIS2_PLACEMENT_3D('',#58221,#45776,#45777);
#37034=AXIS2_PLACEMENT_3D('',#58223,#45778,#45779);
#37035=AXIS2_PLACEMENT_3D('',#58225,#45781,#45782);
#37036=AXIS2_PLACEMENT_3D('',#58228,#45784,#45785);
#37037=AXIS2_PLACEMENT_3D('',#58229,#45786,#45787);
#37038=AXIS2_PLACEMENT_3D('',#58233,#45789,#45790);
#37039=AXIS2_PLACEMENT_3D('',#58235,#45792,#45793);
#37040=AXIS2_PLACEMENT_3D('',#58237,#45794,#45795);
#37041=AXIS2_PLACEMENT_3D('',#58239,#45797,#45798);
#37042=AXIS2_PLACEMENT_3D('',#58242,#45800,#45801);
#37043=AXIS2_PLACEMENT_3D('',#58243,#45802,#45803);
#37044=AXIS2_PLACEMENT_3D('',#58247,#45805,#45806);
#37045=AXIS2_PLACEMENT_3D('',#58249,#45808,#45809);
#37046=AXIS2_PLACEMENT_3D('',#58251,#45810,#45811);
#37047=AXIS2_PLACEMENT_3D('',#58253,#45813,#45814);
#37048=AXIS2_PLACEMENT_3D('',#58256,#45816,#45817);
#37049=AXIS2_PLACEMENT_3D('',#58257,#45818,#45819);
#37050=AXIS2_PLACEMENT_3D('',#58261,#45821,#45822);
#37051=AXIS2_PLACEMENT_3D('',#58263,#45824,#45825);
#37052=AXIS2_PLACEMENT_3D('',#58265,#45826,#45827);
#37053=AXIS2_PLACEMENT_3D('',#58267,#45829,#45830);
#37054=AXIS2_PLACEMENT_3D('',#58270,#45832,#45833);
#37055=AXIS2_PLACEMENT_3D('',#58271,#45834,#45835);
#37056=AXIS2_PLACEMENT_3D('',#58275,#45837,#45838);
#37057=AXIS2_PLACEMENT_3D('',#58277,#45840,#45841);
#37058=AXIS2_PLACEMENT_3D('',#58279,#45842,#45843);
#37059=AXIS2_PLACEMENT_3D('',#58281,#45845,#45846);
#37060=AXIS2_PLACEMENT_3D('',#58284,#45848,#45849);
#37061=AXIS2_PLACEMENT_3D('',#58285,#45850,#45851);
#37062=AXIS2_PLACEMENT_3D('',#58289,#45853,#45854);
#37063=AXIS2_PLACEMENT_3D('',#58291,#45856,#45857);
#37064=AXIS2_PLACEMENT_3D('',#58293,#45858,#45859);
#37065=AXIS2_PLACEMENT_3D('',#58295,#45861,#45862);
#37066=AXIS2_PLACEMENT_3D('',#58298,#45864,#45865);
#37067=AXIS2_PLACEMENT_3D('',#58299,#45866,#45867);
#37068=AXIS2_PLACEMENT_3D('',#58303,#45869,#45870);
#37069=AXIS2_PLACEMENT_3D('',#58305,#45872,#45873);
#37070=AXIS2_PLACEMENT_3D('',#58307,#45874,#45875);
#37071=AXIS2_PLACEMENT_3D('',#58309,#45877,#45878);
#37072=AXIS2_PLACEMENT_3D('',#58312,#45880,#45881);
#37073=AXIS2_PLACEMENT_3D('',#58313,#45882,#45883);
#37074=AXIS2_PLACEMENT_3D('',#58317,#45885,#45886);
#37075=AXIS2_PLACEMENT_3D('',#58319,#45888,#45889);
#37076=AXIS2_PLACEMENT_3D('',#58321,#45890,#45891);
#37077=AXIS2_PLACEMENT_3D('',#58323,#45893,#45894);
#37078=AXIS2_PLACEMENT_3D('',#58326,#45896,#45897);
#37079=AXIS2_PLACEMENT_3D('',#58327,#45898,#45899);
#37080=AXIS2_PLACEMENT_3D('',#58331,#45901,#45902);
#37081=AXIS2_PLACEMENT_3D('',#58333,#45904,#45905);
#37082=AXIS2_PLACEMENT_3D('',#58335,#45906,#45907);
#37083=AXIS2_PLACEMENT_3D('',#58337,#45909,#45910);
#37084=AXIS2_PLACEMENT_3D('',#58340,#45912,#45913);
#37085=AXIS2_PLACEMENT_3D('',#58341,#45914,#45915);
#37086=AXIS2_PLACEMENT_3D('',#58345,#45917,#45918);
#37087=AXIS2_PLACEMENT_3D('',#58347,#45920,#45921);
#37088=AXIS2_PLACEMENT_3D('',#58349,#45922,#45923);
#37089=AXIS2_PLACEMENT_3D('',#58351,#45925,#45926);
#37090=AXIS2_PLACEMENT_3D('',#58354,#45928,#45929);
#37091=AXIS2_PLACEMENT_3D('',#58355,#45930,#45931);
#37092=AXIS2_PLACEMENT_3D('',#58359,#45933,#45934);
#37093=AXIS2_PLACEMENT_3D('',#58361,#45936,#45937);
#37094=AXIS2_PLACEMENT_3D('',#58363,#45938,#45939);
#37095=AXIS2_PLACEMENT_3D('',#58365,#45941,#45942);
#37096=AXIS2_PLACEMENT_3D('',#58368,#45944,#45945);
#37097=AXIS2_PLACEMENT_3D('',#58369,#45946,#45947);
#37098=AXIS2_PLACEMENT_3D('',#58373,#45949,#45950);
#37099=AXIS2_PLACEMENT_3D('',#58375,#45952,#45953);
#37100=AXIS2_PLACEMENT_3D('',#58377,#45954,#45955);
#37101=AXIS2_PLACEMENT_3D('',#58379,#45957,#45958);
#37102=AXIS2_PLACEMENT_3D('',#58382,#45960,#45961);
#37103=AXIS2_PLACEMENT_3D('',#58383,#45962,#45963);
#37104=AXIS2_PLACEMENT_3D('',#58387,#45965,#45966);
#37105=AXIS2_PLACEMENT_3D('',#58389,#45968,#45969);
#37106=AXIS2_PLACEMENT_3D('',#58391,#45970,#45971);
#37107=AXIS2_PLACEMENT_3D('',#58393,#45973,#45974);
#37108=AXIS2_PLACEMENT_3D('',#58396,#45976,#45977);
#37109=AXIS2_PLACEMENT_3D('',#58397,#45978,#45979);
#37110=AXIS2_PLACEMENT_3D('',#58401,#45981,#45982);
#37111=AXIS2_PLACEMENT_3D('',#58403,#45984,#45985);
#37112=AXIS2_PLACEMENT_3D('',#58405,#45986,#45987);
#37113=AXIS2_PLACEMENT_3D('',#58407,#45989,#45990);
#37114=AXIS2_PLACEMENT_3D('',#58410,#45992,#45993);
#37115=AXIS2_PLACEMENT_3D('',#58411,#45994,#45995);
#37116=AXIS2_PLACEMENT_3D('',#58415,#45997,#45998);
#37117=AXIS2_PLACEMENT_3D('',#58417,#46000,#46001);
#37118=AXIS2_PLACEMENT_3D('',#58419,#46002,#46003);
#37119=AXIS2_PLACEMENT_3D('',#58421,#46005,#46006);
#37120=AXIS2_PLACEMENT_3D('',#58424,#46008,#46009);
#37121=AXIS2_PLACEMENT_3D('',#58425,#46010,#46011);
#37122=AXIS2_PLACEMENT_3D('',#58429,#46013,#46014);
#37123=AXIS2_PLACEMENT_3D('',#58431,#46016,#46017);
#37124=AXIS2_PLACEMENT_3D('',#58433,#46018,#46019);
#37125=AXIS2_PLACEMENT_3D('',#58435,#46021,#46022);
#37126=AXIS2_PLACEMENT_3D('',#58438,#46024,#46025);
#37127=AXIS2_PLACEMENT_3D('',#58439,#46026,#46027);
#37128=AXIS2_PLACEMENT_3D('',#58443,#46029,#46030);
#37129=AXIS2_PLACEMENT_3D('',#58445,#46032,#46033);
#37130=AXIS2_PLACEMENT_3D('',#58447,#46034,#46035);
#37131=AXIS2_PLACEMENT_3D('',#58449,#46037,#46038);
#37132=AXIS2_PLACEMENT_3D('',#58452,#46040,#46041);
#37133=AXIS2_PLACEMENT_3D('',#58453,#46042,#46043);
#37134=AXIS2_PLACEMENT_3D('',#58457,#46045,#46046);
#37135=AXIS2_PLACEMENT_3D('',#58459,#46048,#46049);
#37136=AXIS2_PLACEMENT_3D('',#58461,#46050,#46051);
#37137=AXIS2_PLACEMENT_3D('',#58463,#46053,#46054);
#37138=AXIS2_PLACEMENT_3D('',#58466,#46056,#46057);
#37139=AXIS2_PLACEMENT_3D('',#58467,#46058,#46059);
#37140=AXIS2_PLACEMENT_3D('',#58471,#46061,#46062);
#37141=AXIS2_PLACEMENT_3D('',#58473,#46064,#46065);
#37142=AXIS2_PLACEMENT_3D('',#58475,#46066,#46067);
#37143=AXIS2_PLACEMENT_3D('',#58477,#46069,#46070);
#37144=AXIS2_PLACEMENT_3D('',#58480,#46072,#46073);
#37145=AXIS2_PLACEMENT_3D('',#58481,#46074,#46075);
#37146=AXIS2_PLACEMENT_3D('',#58485,#46077,#46078);
#37147=AXIS2_PLACEMENT_3D('',#58487,#46080,#46081);
#37148=AXIS2_PLACEMENT_3D('',#58489,#46082,#46083);
#37149=AXIS2_PLACEMENT_3D('',#58491,#46085,#46086);
#37150=AXIS2_PLACEMENT_3D('',#58494,#46088,#46089);
#37151=AXIS2_PLACEMENT_3D('',#58495,#46090,#46091);
#37152=AXIS2_PLACEMENT_3D('',#58499,#46093,#46094);
#37153=AXIS2_PLACEMENT_3D('',#58501,#46096,#46097);
#37154=AXIS2_PLACEMENT_3D('',#58503,#46098,#46099);
#37155=AXIS2_PLACEMENT_3D('',#58505,#46101,#46102);
#37156=AXIS2_PLACEMENT_3D('',#58508,#46104,#46105);
#37157=AXIS2_PLACEMENT_3D('',#58509,#46106,#46107);
#37158=AXIS2_PLACEMENT_3D('',#58511,#46108,#46109);
#37159=AXIS2_PLACEMENT_3D('',#58513,#46111,#46112);
#37160=AXIS2_PLACEMENT_3D('',#58514,#46113,#46114);
#37161=AXIS2_PLACEMENT_3D('',#58515,#46115,#46116);
#37162=AXIS2_PLACEMENT_3D('',#58516,#46117,#46118);
#37163=AXIS2_PLACEMENT_3D('',#58517,#46119,#46120);
#37164=AXIS2_PLACEMENT_3D('',#58518,#46121,#46122);
#37165=AXIS2_PLACEMENT_3D('',#58519,#46123,#46124);
#37166=AXIS2_PLACEMENT_3D('',#58520,#46125,#46126);
#37167=AXIS2_PLACEMENT_3D('',#58521,#46127,#46128);
#37168=AXIS2_PLACEMENT_3D('',#58522,#46129,#46130);
#37169=AXIS2_PLACEMENT_3D('',#58523,#46131,#46132);
#37170=AXIS2_PLACEMENT_3D('',#58524,#46133,#46134);
#37171=AXIS2_PLACEMENT_3D('',#58525,#46135,#46136);
#37172=AXIS2_PLACEMENT_3D('',#58526,#46137,#46138);
#37173=AXIS2_PLACEMENT_3D('',#58527,#46139,#46140);
#37174=AXIS2_PLACEMENT_3D('',#58528,#46141,#46142);
#37175=AXIS2_PLACEMENT_3D('',#58529,#46143,#46144);
#37176=AXIS2_PLACEMENT_3D('',#58530,#46145,#46146);
#37177=AXIS2_PLACEMENT_3D('',#58531,#46147,#46148);
#37178=AXIS2_PLACEMENT_3D('',#58532,#46149,#46150);
#37179=AXIS2_PLACEMENT_3D('',#58533,#46151,#46152);
#37180=AXIS2_PLACEMENT_3D('',#58534,#46153,#46154);
#37181=AXIS2_PLACEMENT_3D('',#58535,#46155,#46156);
#37182=AXIS2_PLACEMENT_3D('',#58536,#46157,#46158);
#37183=AXIS2_PLACEMENT_3D('',#58537,#46159,#46160);
#37184=AXIS2_PLACEMENT_3D('',#58538,#46161,#46162);
#37185=AXIS2_PLACEMENT_3D('',#58539,#46163,#46164);
#37186=AXIS2_PLACEMENT_3D('',#58540,#46165,#46166);
#37187=AXIS2_PLACEMENT_3D('',#58541,#46167,#46168);
#37188=AXIS2_PLACEMENT_3D('',#58542,#46169,#46170);
#37189=AXIS2_PLACEMENT_3D('',#58543,#46171,#46172);
#37190=AXIS2_PLACEMENT_3D('',#58544,#46173,#46174);
#37191=AXIS2_PLACEMENT_3D('',#58545,#46175,#46176);
#37192=AXIS2_PLACEMENT_3D('',#58546,#46177,#46178);
#37193=AXIS2_PLACEMENT_3D('',#58547,#46179,#46180);
#37194=AXIS2_PLACEMENT_3D('',#58548,#46181,#46182);
#37195=AXIS2_PLACEMENT_3D('',#58549,#46183,#46184);
#37196=AXIS2_PLACEMENT_3D('',#58550,#46185,#46186);
#37197=AXIS2_PLACEMENT_3D('',#58551,#46187,#46188);
#37198=AXIS2_PLACEMENT_3D('',#58552,#46189,#46190);
#37199=AXIS2_PLACEMENT_3D('',#58553,#46191,#46192);
#37200=AXIS2_PLACEMENT_3D('',#58554,#46193,#46194);
#37201=AXIS2_PLACEMENT_3D('',#58555,#46195,#46196);
#37202=AXIS2_PLACEMENT_3D('',#58556,#46197,#46198);
#37203=AXIS2_PLACEMENT_3D('',#58557,#46199,#46200);
#37204=AXIS2_PLACEMENT_3D('',#58558,#46201,#46202);
#37205=AXIS2_PLACEMENT_3D('',#58559,#46203,#46204);
#37206=AXIS2_PLACEMENT_3D('',#58560,#46205,#46206);
#37207=AXIS2_PLACEMENT_3D('',#58561,#46207,#46208);
#37208=AXIS2_PLACEMENT_3D('',#58562,#46209,#46210);
#37209=AXIS2_PLACEMENT_3D('',#58563,#46211,#46212);
#37210=AXIS2_PLACEMENT_3D('',#58564,#46213,#46214);
#37211=AXIS2_PLACEMENT_3D('',#58565,#46215,#46216);
#37212=AXIS2_PLACEMENT_3D('',#58566,#46217,#46218);
#37213=AXIS2_PLACEMENT_3D('',#58567,#46219,#46220);
#37214=AXIS2_PLACEMENT_3D('',#58568,#46221,#46222);
#37215=AXIS2_PLACEMENT_3D('',#58569,#46223,#46224);
#37216=AXIS2_PLACEMENT_3D('',#58570,#46225,#46226);
#37217=AXIS2_PLACEMENT_3D('',#58571,#46227,#46228);
#37218=AXIS2_PLACEMENT_3D('',#58572,#46229,#46230);
#37219=AXIS2_PLACEMENT_3D('',#58573,#46231,#46232);
#37220=AXIS2_PLACEMENT_3D('',#58574,#46233,#46234);
#37221=AXIS2_PLACEMENT_3D('',#58575,#46235,#46236);
#37222=AXIS2_PLACEMENT_3D('',#58576,#46237,#46238);
#37223=AXIS2_PLACEMENT_3D('',#58577,#46239,#46240);
#37224=AXIS2_PLACEMENT_3D('',#58578,#46241,#46242);
#37225=AXIS2_PLACEMENT_3D('',#58579,#46243,#46244);
#37226=AXIS2_PLACEMENT_3D('',#58580,#46245,#46246);
#37227=AXIS2_PLACEMENT_3D('',#58581,#46247,#46248);
#37228=AXIS2_PLACEMENT_3D('',#58582,#46249,#46250);
#37229=AXIS2_PLACEMENT_3D('',#58583,#46251,#46252);
#37230=AXIS2_PLACEMENT_3D('',#58584,#46253,#46254);
#37231=AXIS2_PLACEMENT_3D('',#58585,#46255,#46256);
#37232=AXIS2_PLACEMENT_3D('',#58586,#46257,#46258);
#37233=AXIS2_PLACEMENT_3D('',#58587,#46259,#46260);
#37234=AXIS2_PLACEMENT_3D('',#58588,#46261,#46262);
#37235=AXIS2_PLACEMENT_3D('',#58589,#46263,#46264);
#37236=AXIS2_PLACEMENT_3D('',#58593,#46266,#46267);
#37237=AXIS2_PLACEMENT_3D('',#58595,#46269,#46270);
#37238=AXIS2_PLACEMENT_3D('',#58597,#46271,#46272);
#37239=AXIS2_PLACEMENT_3D('',#58599,#46274,#46275);
#37240=AXIS2_PLACEMENT_3D('',#58600,#46276,#46277);
#37241=AXIS2_PLACEMENT_3D('',#58601,#46278,#46279);
#37242=AXIS2_PLACEMENT_3D('',#58602,#46280,#46281);
#37243=AXIS2_PLACEMENT_3D('',#58603,#46282,#46283);
#45113=DIRECTION('axis',(0.,0.,1.));
#45114=DIRECTION('refdir',(1.,0.,0.));
#45115=DIRECTION('center_axis',(3.66113466765123E-16,1.,-5.66153840231349E-16));
#45116=DIRECTION('ref_axis',(0.996957691137886,-2.96059473233375E-16,0.0779446090567888));
#45117=DIRECTION('center_axis',(-3.66113466765123E-16,-1.,5.66153840231349E-16));
#45118=DIRECTION('ref_axis',(-0.996957691137886,3.20870996777813E-16,-0.0779446090567869));
#45119=DIRECTION('center_axis',(-0.0779446090567859,5.92967996423326E-16,
0.996957691137886));
#45120=DIRECTION('ref_axis',(-0.996957691137886,3.33066907387547E-16,-0.0779446090567859));
#45121=DIRECTION('center_axis',(3.66113466765123E-16,1.,-5.66153840231349E-16));
#45122=DIRECTION('ref_axis',(-0.996957691137886,3.20870996777813E-16,-0.0779446090567869));
#45123=DIRECTION('center_axis',(3.66113466765123E-16,1.,-5.66153840231349E-16));
#45124=DIRECTION('ref_axis',(-0.996957691137886,3.20870996777813E-16,-0.0779446090567869));
#45125=DIRECTION('center_axis',(3.66113466765123E-16,1.,-5.66153840231349E-16));
#45126=DIRECTION('ref_axis',(-0.996957691137886,3.20870996777813E-16,-0.0779446090567869));
#45127=DIRECTION('',(-3.66113466765123E-16,-1.,5.66153840231349E-16));
#45128=DIRECTION('center_axis',(-3.66113466765123E-16,-1.,5.66153840231349E-16));
#45129=DIRECTION('ref_axis',(-0.996957691137886,3.20870996777813E-16,-0.0779446090567869));
#45130=DIRECTION('center_axis',(3.66113466765123E-16,1.,-5.66153840231349E-16));
#45131=DIRECTION('ref_axis',(0.996957691137886,-3.20870996777813E-16,0.0779446090567869));
#45132=DIRECTION('',(0.0779446090567869,-5.92967996423326E-16,-0.996957691137886));
#45133=DIRECTION('',(0.996957691137886,-3.20870996777813E-16,0.0779446090567869));
#45134=DIRECTION('',(-0.0779446090567869,5.92967996423326E-16,0.996957691137886));
#45135=DIRECTION('center_axis',(-3.66113466765123E-16,-1.,5.66153840231349E-16));
#45136=DIRECTION('ref_axis',(0.327345662251861,4.15115746948114E-16,0.944904660484268));
#45137=DIRECTION('center_axis',(-3.66113466765123E-16,-1.,5.66153840231349E-16));
#45138=DIRECTION('ref_axis',(-0.996957691137886,3.1347473636475E-16,-0.0779446090567884));
#45139=DIRECTION('center_axis',(3.66113466765123E-16,1.,-5.66153840231349E-16));
#45140=DIRECTION('ref_axis',(-0.996957691137886,3.20870996777813E-16,-0.0779446090567869));
#45141=DIRECTION('center_axis',(0.077944609056788,-5.92967996423326E-16,
-0.996957691137886));
#45142=DIRECTION('ref_axis',(0.996957691137886,-3.26536183713281E-16,0.077944609056788));
#45143=DIRECTION('center_axis',(-3.66113466765123E-16,-1.,5.66153840231349E-16));
#45144=DIRECTION('ref_axis',(-0.996957691137886,3.20870996777813E-16,-0.0779446090567869));
#45145=DIRECTION('center_axis',(3.66113466765123E-16,1.,-5.66153840231349E-16));
#45146=DIRECTION('ref_axis',(-0.993453242215613,2.99039498345089E-16,-0.114239465734422));
#45147=DIRECTION('center_axis',(3.66113466765123E-16,1.,-5.66153840231349E-16));
#45148=DIRECTION('ref_axis',(-0.176304286675074,-4.92738071143036E-16,-0.984335714327177));
#45149=DIRECTION('center_axis',(3.66113466765123E-16,1.,-5.66153840231349E-16));
#45150=DIRECTION('ref_axis',(0.798717078866636,-6.33079672938476E-16,-0.601706762407361));
#45151=DIRECTION('center_axis',(-3.66113466765123E-16,-1.,5.66153840231349E-16));
#45152=DIRECTION('ref_axis',(-0.996957691137886,3.20870996777813E-16,-0.0779446090567869));
#45153=DIRECTION('center_axis',(3.66113466765123E-16,1.,-5.66153840231349E-16));
#45154=DIRECTION('ref_axis',(-0.999093173971444,3.89886789042682E-16,0.0425773381467764));
#45155=DIRECTION('center_axis',(3.66113466765123E-16,1.,-5.66153840231349E-16));
#45156=DIRECTION('ref_axis',(-0.328117719236679,-4.14681459743577E-16,-0.944636841502024));
#45157=DIRECTION('center_axis',(3.66113466765123E-16,1.,-5.66153840231349E-16));
#45158=DIRECTION('ref_axis',(0.694755870742498,-6.61563157380586E-16,-0.719245632637998));
#45159=DIRECTION('center_axis',(-3.66113466765123E-16,-1.,5.66153840231349E-16));
#45160=DIRECTION('ref_axis',(-0.996957691137886,3.20870996777813E-16,-0.0779446090567869));
#45161=DIRECTION('center_axis',(3.66113466765123E-16,1.,-5.66153840231349E-16));
#45162=DIRECTION('ref_axis',(-0.980132115983957,4.71133773033976E-16,0.198345746656716));
#45163=DIRECTION('center_axis',(3.66113466765123E-16,1.,-5.66153840231349E-16));
#45164=DIRECTION('ref_axis',(-0.471851804590399,-3.26414014556371E-16,-0.881677874569156));
#45165=DIRECTION('center_axis',(3.66113466765123E-16,1.,-5.66153840231349E-16));
#45166=DIRECTION('ref_axis',(0.573687467318141,-6.73756761285746E-16,-0.819074288353686));
#45167=DIRECTION('center_axis',(-3.66113466765123E-16,-1.,5.66153840231349E-16));
#45168=DIRECTION('ref_axis',(-0.996957691137886,3.20870996777813E-16,-0.0779446090567869));
#45169=DIRECTION('center_axis',(3.66113466765123E-16,1.,-5.66153840231349E-16));
#45170=DIRECTION('ref_axis',(-0.937036952428947,5.40779879929828E-16,0.349230224612176));
#45171=DIRECTION('center_axis',(3.66113466765123E-16,1.,-5.66153840231349E-16));
#45172=DIRECTION('ref_axis',(-0.603967332528746,-2.30109173024781E-16,-0.797009072243291));
#45173=DIRECTION('center_axis',(3.66113466765123E-16,1.,-5.66153840231349E-16));
#45174=DIRECTION('ref_axis',(0.438492974488865,-6.6936023765756E-16,-0.898734616738394));
#45175=DIRECTION('center_axis',(-3.66113466765123E-16,-1.,5.66153840231349E-16));
#45176=DIRECTION('ref_axis',(-0.996957691137886,3.20870996777813E-16,-0.0779446090567869));
#45177=DIRECTION('center_axis',(3.66113466765123E-16,1.,-5.66153840231349E-16));
#45178=DIRECTION('ref_axis',(-0.870868829257786,5.97110191436282E-16,0.491515495409018));
#45179=DIRECTION('center_axis',(3.66113466765123E-16,1.,-5.66153840231349E-16));
#45180=DIRECTION('ref_axis',(-0.721211180287579,-1.28138279964759E-16,-0.692715261437336));
#45181=DIRECTION('center_axis',(3.66113466765123E-16,1.,-5.66153840231349E-16));
#45182=DIRECTION('ref_axis',(0.292501329352925,-6.48481843498979E-16,-0.956265116129817));
#45183=DIRECTION('center_axis',(-3.66113466765123E-16,-1.,5.66153840231349E-16));
#45184=DIRECTION('ref_axis',(-0.996957691137886,3.20870996777813E-16,-0.0779446090567869));
#45185=DIRECTION('center_axis',(3.66113466765123E-16,1.,-5.66153840231349E-16));
#45186=DIRECTION('ref_axis',(-0.78325702526236,6.38737668334465E-16,0.621698023462484));
#45187=DIRECTION('center_axis',(3.66113466765123E-16,1.,-5.66153840231349E-16));
#45188=DIRECTION('ref_axis',(-0.820696415225053,-2.30121971854362E-17,-0.571364501904649));
#45189=DIRECTION('center_axis',(3.66113466765123E-16,1.,-5.66153840231349E-16));
#45190=DIRECTION('ref_axis',(0.139307330732061,-6.11635674165605E-16,-0.990249194700156));
#45191=DIRECTION('center_axis',(-3.66113466765123E-16,-1.,5.66153840231349E-16));
#45192=DIRECTION('ref_axis',(-0.996957691137886,3.20870996777813E-16,-0.0779446090567869));
#45193=DIRECTION('center_axis',(3.66113466765123E-16,1.,-5.66153840231349E-16));
#45194=DIRECTION('ref_axis',(-0.676358833823941,6.64637303989468E-16,0.736572282880858));
#45195=DIRECTION('center_axis',(3.66113466765123E-16,1.,-5.66153840231349E-16));
#45196=DIRECTION('ref_axis',(-0.899973380684442,8.26805222616965E-17,-0.435944852085004));
#45197=DIRECTION('center_axis',(3.66113466765123E-16,1.,-5.66153840231349E-16));
#45198=DIRECTION('ref_axis',(-0.0173168767059515,-5.5972900463185E-16,-0.999850051648321));
#45199=DIRECTION('center_axis',(-3.66113466765123E-16,-1.,5.66153840231349E-16));
#45200=DIRECTION('ref_axis',(-0.996957691137886,3.20870996777813E-16,-0.0779446090567869));
#45201=DIRECTION('center_axis',(3.66113466765123E-16,1.,-5.66153840231349E-16));
#45202=DIRECTION('ref_axis',(-0.552806443190503,6.74171363415503E-16,0.833309688151449));
#45203=DIRECTION('center_axis',(3.66113466765123E-16,1.,-5.66153840231349E-16));
#45204=DIRECTION('ref_axis',(-0.957090014670973,1.86337372849825E-16,-0.289790793189011));
#45205=DIRECTION('center_axis',(3.66113466765123E-16,1.,-5.66153840231349E-16));
#45206=DIRECTION('ref_axis',(-0.173514685168044,-4.94039949369995E-16,-0.98483128201283));
#45207=DIRECTION('center_axis',(-3.66113466765123E-16,-1.,5.66153840231349E-16));
#45208=DIRECTION('ref_axis',(-0.996957691137886,3.20870996777813E-16,-0.0779446090567869));
#45209=DIRECTION('center_axis',(3.66113466765123E-16,1.,-5.66153840231349E-16));
#45210=DIRECTION('ref_axis',(-0.415642123266314,6.67105086427771E-16,0.909528243303456));
#45211=DIRECTION('center_axis',(3.66113466765123E-16,1.,-5.66153840231349E-16));
#45212=DIRECTION('ref_axis',(-0.990639916096657,2.85405978900106E-16,-0.136501123204203));
#45213=DIRECTION('center_axis',(3.66113466765123E-16,1.,-5.66153840231349E-16));
#45214=DIRECTION('ref_axis',(-0.325439986219075,-4.16185990930063E-16,-0.945562697746547));
#45215=DIRECTION('center_axis',(-3.66113466765123E-16,-1.,5.66153840231349E-16));
#45216=DIRECTION('ref_axis',(-0.996957691137886,3.20870996777813E-16,-0.0779446090567869));
#45217=DIRECTION('center_axis',(3.66113466765123E-16,1.,-5.66153840231349E-16));
#45218=DIRECTION('ref_axis',(-0.268243314830189,6.43612468217339E-16,0.963351194554152));
#45219=DIRECTION('center_axis',(3.66113466765123E-16,1.,-5.66153840231349E-16));
#45220=DIRECTION('ref_axis',(-0.999796975042654,3.77446942541727E-16,0.0201496574551479));
#45221=DIRECTION('center_axis',(3.66113466765123E-16,1.,-5.66153840231349E-16));
#45222=DIRECTION('ref_axis',(-0.469351874736002,-3.28084152151318E-16,-0.883011221719068));
#45223=DIRECTION('center_axis',(-3.66113466765123E-16,-1.,5.66153840231349E-16));
#45224=DIRECTION('ref_axis',(-0.996957691137886,3.20870996777813E-16,-0.0779446090567869));
#45225=DIRECTION('center_axis',(3.66113466765123E-16,1.,-5.66153840231349E-16));
#45226=DIRECTION('ref_axis',(-0.114239465734422,6.04271975012079E-16,0.993453242215613));
#45227=DIRECTION('center_axis',(3.66113466765123E-16,1.,-5.66153840231349E-16));
#45228=DIRECTION('ref_axis',(-0.984335714327177,4.60193909783388E-16,0.176304286675074));
#45229=DIRECTION('center_axis',(3.66113466765123E-16,1.,-5.66153840231349E-16));
#45230=DIRECTION('ref_axis',(-0.601706762407361,-2.31903792697734E-16,-0.798717078866636));
#45231=DIRECTION('center_axis',(-3.66113466765123E-16,-1.,5.66153840231349E-16));
#45232=DIRECTION('ref_axis',(-0.996957691137886,3.20870996777813E-16,-0.0779446090567869));
#45233=DIRECTION('center_axis',(3.66113466765123E-16,1.,-5.66153840231349E-16));
#45234=DIRECTION('ref_axis',(0.0425773381467764,5.50052300318313E-16,0.999093173971444));
#45235=DIRECTION('center_axis',(3.66113466765123E-16,1.,-5.66153840231349E-16));
#45236=DIRECTION('ref_axis',(-0.944636841502024,5.31609375670159E-16,0.328117719236679));
#45237=DIRECTION('center_axis',(3.66113466765123E-16,1.,-5.66153840231349E-16));
#45238=DIRECTION('ref_axis',(-0.719245632637998,-1.30013192223369E-16,-0.694755870742498));
#45239=DIRECTION('center_axis',(-3.66113466765123E-16,-1.,5.66153840231349E-16));
#45240=DIRECTION('ref_axis',(-0.996957691137886,3.20870996777813E-16,-0.0779446090567869));
#45241=DIRECTION('center_axis',(3.66113466765123E-16,1.,-5.66153840231349E-16));
#45242=DIRECTION('ref_axis',(0.198345746656716,4.82288512471788E-16,0.980132115983957));
#45243=DIRECTION('center_axis',(3.66113466765123E-16,1.,-5.66153840231349E-16));
#45244=DIRECTION('ref_axis',(-0.881677874569156,5.89934854417565E-16,0.471851804590399));
#45245=DIRECTION('center_axis',(3.66113466765123E-16,1.,-5.66153840231349E-16));
#45246=DIRECTION('ref_axis',(-0.819074288353686,-2.49212354674179E-17,-0.573687467318141));
#45247=DIRECTION('center_axis',(-3.66113466765123E-16,-1.,5.66153840231349E-16));
#45248=DIRECTION('ref_axis',(-0.996957691137886,3.20870996777813E-16,-0.0779446090567869));
#45249=DIRECTION('center_axis',(3.66113466765123E-16,1.,-5.66153840231349E-16));
#45250=DIRECTION('ref_axis',(0.349230224612176,4.02649180824402E-16,0.937036952428947));
#45251=DIRECTION('center_axis',(3.66113466765123E-16,1.,-5.66153840231349E-16));
#45252=DIRECTION('ref_axis',(-0.797009072243291,6.33734179167679E-16,0.603967332528746));
#45253=DIRECTION('center_axis',(3.66113466765123E-16,1.,-5.66153840231349E-16));
#45254=DIRECTION('ref_axis',(-0.898734616738394,8.07843648145798E-17,-0.438492974488865));
#45255=DIRECTION('center_axis',(-3.66113466765123E-16,-1.,5.66153840231349E-16));
#45256=DIRECTION('ref_axis',(-0.996957691137886,3.20870996777813E-16,-0.0779446090567869));
#45257=DIRECTION('center_axis',(3.66113466765123E-16,1.,-5.66153840231349E-16));
#45258=DIRECTION('ref_axis',(0.491515495409017,3.13095290029103E-16,0.870868829257787));
#45259=DIRECTION('center_axis',(3.66113466765123E-16,1.,-5.66153840231349E-16));
#45260=DIRECTION('ref_axis',(-0.692715261437337,6.61928865183528E-16,0.721211180287579));
#45261=DIRECTION('center_axis',(3.66113466765123E-16,1.,-5.66153840231349E-16));
#45262=DIRECTION('ref_axis',(-0.956265116129817,1.84500785926907E-16,-0.292501329352925));
#45263=DIRECTION('center_axis',(-3.66113466765123E-16,-1.,5.66153840231349E-16));
#45264=DIRECTION('ref_axis',(-0.996957691137886,3.20870996777813E-16,-0.0779446090567869));
#45265=DIRECTION('center_axis',(3.66113466765123E-16,1.,-5.66153840231349E-16));
#45266=DIRECTION('ref_axis',(0.621698023462484,2.15831954089593E-16,0.78325702526236));
#45267=DIRECTION('center_axis',(3.66113466765123E-16,1.,-5.66153840231349E-16));
#45268=DIRECTION('ref_axis',(-0.571364501904649,6.73824665722604E-16,0.820696415225053));
#45269=DIRECTION('center_axis',(3.66113466765123E-16,1.,-5.66153840231349E-16));
#45270=DIRECTION('ref_axis',(-0.990249194700156,2.83674185366711E-16,-0.13930733073206));
#45271=DIRECTION('center_axis',(-3.66113466765123E-16,-1.,5.66153840231349E-16));
#45272=DIRECTION('ref_axis',(-0.996957691137886,3.20870996777813E-16,-0.0779446090567869));
#45273=DIRECTION('center_axis',(3.66113466765123E-16,1.,-5.66153840231349E-16));
#45274=DIRECTION('ref_axis',(0.736572282880858,1.1325411913521E-16,0.676358833823941));
#45275=DIRECTION('center_axis',(3.66113466765123E-16,1.,-5.66153840231349E-16));
#45276=DIRECTION('ref_axis',(-0.435944852085004,6.69128666695736E-16,0.899973380684442));
#45277=DIRECTION('center_axis',(3.66113466765123E-16,1.,-5.66153840231349E-16));
#45278=DIRECTION('ref_axis',(-0.999850051648321,3.75862584902141E-16,0.0173168767059515));
#45279=DIRECTION('center_axis',(-3.66113466765123E-16,-1.,5.66153840231349E-16));
#45280=DIRECTION('ref_axis',(-0.996957691137886,3.20870996777813E-16,-0.0779446090567869));
#45281=DIRECTION('center_axis',(3.66113466765123E-16,1.,-5.66153840231349E-16));
#45282=DIRECTION('ref_axis',(0.833309688151449,7.88759189884587E-18,0.552806443190503));
#45283=DIRECTION('center_axis',(3.66113466765123E-16,1.,-5.66153840231349E-16));
#45284=DIRECTION('ref_axis',(-0.289790793189011,6.47956499184093E-16,0.957090014670973));
#45285=DIRECTION('center_axis',(3.66113466765123E-16,1.,-5.66153840231349E-16));
#45286=DIRECTION('ref_axis',(-0.98483128201283,4.5879600018088E-16,0.173514685168044));
#45287=DIRECTION('center_axis',(-3.66113466765123E-16,-1.,5.66153840231349E-16));
#45288=DIRECTION('ref_axis',(-0.996957691137886,3.20870996777813E-16,-0.0779446090567869));
#45289=DIRECTION('center_axis',(3.66113466765123E-16,1.,-5.66153840231349E-16));
#45290=DIRECTION('ref_axis',(0.909528243303456,-9.76731540274849E-17,0.415642123266314));
#45291=DIRECTION('center_axis',(3.66113466765123E-16,1.,-5.66153840231349E-16));
#45292=DIRECTION('ref_axis',(-0.136501123204203,6.10829492218208E-16,0.990639916096657));
#45293=DIRECTION('center_axis',(3.66113466765123E-16,1.,-5.66153840231349E-16));
#45294=DIRECTION('ref_axis',(-0.945562697746547,5.30432335278537E-16,0.325439986219075));
#45295=DIRECTION('center_axis',(-3.66113466765123E-16,-1.,5.66153840231349E-16));
#45296=DIRECTION('ref_axis',(-0.996957691137886,3.20870996777813E-16,-0.0779446090567869));
#45297=DIRECTION('center_axis',(3.66113466765123E-16,1.,-5.66153840231349E-16));
#45298=DIRECTION('ref_axis',(0.963351194554152,-2.00828862743045E-16,0.268243314830189));
#45299=DIRECTION('center_axis',(3.66113466765123E-16,1.,-5.66153840231349E-16));
#45300=DIRECTION('ref_axis',(0.0201496574551478,5.58661835927051E-16,0.999796975042654));
#45301=DIRECTION('center_axis',(3.66113466765123E-16,1.,-5.66153840231349E-16));
#45302=DIRECTION('ref_axis',(-0.883011221719068,5.89007665877645E-16,0.469351874736002));
#45303=DIRECTION('center_axis',(-3.66113466765123E-16,-1.,5.66153840231349E-16));
#45304=DIRECTION('ref_axis',(-0.996957691137886,3.20870996777813E-16,-0.0779446090567869));
#45305=DIRECTION('center_axis',(3.66113466765123E-16,1.,-5.66153840231349E-16));
#45306=DIRECTION('ref_axis',(0.993453242215613,-2.99039498345089E-16,0.114239465734422));
#45307=DIRECTION('center_axis',(3.66113466765123E-16,1.,-5.66153840231349E-16));
#45308=DIRECTION('ref_axis',(0.176304286675074,4.92738071143036E-16,0.984335714327177));
#45309=DIRECTION('center_axis',(3.66113466765123E-16,1.,-5.66153840231349E-16));
#45310=DIRECTION('ref_axis',(-0.798717078866636,6.33079672938476E-16,0.601706762407361));
#45311=DIRECTION('center_axis',(-3.66113466765123E-16,-1.,5.66153840231349E-16));
#45312=DIRECTION('ref_axis',(-0.996957691137886,3.20870996777813E-16,-0.0779446090567869));
#45313=DIRECTION('center_axis',(3.66113466765123E-16,1.,-5.66153840231349E-16));
#45314=DIRECTION('ref_axis',(0.999093173971444,-3.89886789042682E-16,-0.0425773381467764));
#45315=DIRECTION('center_axis',(3.66113466765123E-16,1.,-5.66153840231349E-16));
#45316=DIRECTION('ref_axis',(0.328117719236679,4.14681459743577E-16,0.944636841502024));
#45317=DIRECTION('center_axis',(3.66113466765123E-16,1.,-5.66153840231349E-16));
#45318=DIRECTION('ref_axis',(-0.694755870742498,6.61563157380586E-16,0.719245632637998));
#45319=DIRECTION('center_axis',(-3.66113466765123E-16,-1.,5.66153840231349E-16));
#45320=DIRECTION('ref_axis',(-0.996957691137886,3.20870996777813E-16,-0.0779446090567869));
#45321=DIRECTION('center_axis',(3.66113466765123E-16,1.,-5.66153840231349E-16));
#45322=DIRECTION('ref_axis',(0.980132115983957,-4.71133773033976E-16,-0.198345746656716));
#45323=DIRECTION('center_axis',(3.66113466765123E-16,1.,-5.66153840231349E-16));
#45324=DIRECTION('ref_axis',(0.471851804590399,3.26414014556371E-16,0.881677874569156));
#45325=DIRECTION('center_axis',(3.66113466765123E-16,1.,-5.66153840231349E-16));
#45326=DIRECTION('ref_axis',(-0.573687467318141,6.73756761285746E-16,0.819074288353686));
#45327=DIRECTION('center_axis',(-3.66113466765123E-16,-1.,5.66153840231349E-16));
#45328=DIRECTION('ref_axis',(-0.996957691137886,3.20870996777813E-16,-0.0779446090567869));
#45329=DIRECTION('center_axis',(3.66113466765123E-16,1.,-5.66153840231349E-16));
#45330=DIRECTION('ref_axis',(0.937036952428947,-5.40779879929828E-16,-0.349230224612176));
#45331=DIRECTION('center_axis',(3.66113466765123E-16,1.,-5.66153840231349E-16));
#45332=DIRECTION('ref_axis',(0.603967332528746,2.30109173024781E-16,0.797009072243291));
#45333=DIRECTION('center_axis',(3.66113466765123E-16,1.,-5.66153840231349E-16));
#45334=DIRECTION('ref_axis',(-0.438492974488865,6.6936023765756E-16,0.898734616738394));
#45335=DIRECTION('center_axis',(-3.66113466765123E-16,-1.,5.66153840231349E-16));
#45336=DIRECTION('ref_axis',(-0.996957691137886,3.20870996777813E-16,-0.0779446090567869));
#45337=DIRECTION('center_axis',(3.66113466765123E-16,1.,-5.66153840231349E-16));
#45338=DIRECTION('ref_axis',(0.870868829257786,-5.97110191436282E-16,-0.491515495409018));
#45339=DIRECTION('center_axis',(3.66113466765123E-16,1.,-5.66153840231349E-16));
#45340=DIRECTION('ref_axis',(0.721211180287579,1.2813827996476E-16,0.692715261437337));
#45341=DIRECTION('center_axis',(3.66113466765123E-16,1.,-5.66153840231349E-16));
#45342=DIRECTION('ref_axis',(-0.292501329352925,6.48481843498979E-16,0.956265116129817));
#45343=DIRECTION('center_axis',(-3.66113466765123E-16,-1.,5.66153840231349E-16));
#45344=DIRECTION('ref_axis',(-0.996957691137886,3.20870996777813E-16,-0.0779446090567869));
#45345=DIRECTION('center_axis',(3.66113466765123E-16,1.,-5.66153840231349E-16));
#45346=DIRECTION('ref_axis',(0.78325702526236,-6.38737668334465E-16,-0.621698023462484));
#45347=DIRECTION('center_axis',(3.66113466765123E-16,1.,-5.66153840231349E-16));
#45348=DIRECTION('ref_axis',(0.820696415225053,2.30121971854362E-17,0.571364501904649));
#45349=DIRECTION('center_axis',(3.66113466765123E-16,1.,-5.66153840231349E-16));
#45350=DIRECTION('ref_axis',(-0.13930733073206,6.11635674165605E-16,0.990249194700156));
#45351=DIRECTION('center_axis',(-3.66113466765123E-16,-1.,5.66153840231349E-16));
#45352=DIRECTION('ref_axis',(-0.996957691137886,3.20870996777813E-16,-0.0779446090567869));
#45353=DIRECTION('center_axis',(3.66113466765123E-16,1.,-5.66153840231349E-16));
#45354=DIRECTION('ref_axis',(0.676358833823941,-6.64637303989468E-16,-0.736572282880858));
#45355=DIRECTION('center_axis',(3.66113466765123E-16,1.,-5.66153840231349E-16));
#45356=DIRECTION('ref_axis',(0.899973380684442,-8.26805222616965E-17,0.435944852085004));
#45357=DIRECTION('center_axis',(3.66113466765123E-16,1.,-5.66153840231349E-16));
#45358=DIRECTION('ref_axis',(0.0173168767059515,5.5972900463185E-16,0.999850051648321));
#45359=DIRECTION('center_axis',(-3.66113466765123E-16,-1.,5.66153840231349E-16));
#45360=DIRECTION('ref_axis',(-0.996957691137886,3.20870996777813E-16,-0.0779446090567869));
#45361=DIRECTION('center_axis',(3.66113466765123E-16,1.,-5.66153840231349E-16));
#45362=DIRECTION('ref_axis',(0.552806443190503,-6.74171363415503E-16,-0.833309688151449));
#45363=DIRECTION('center_axis',(3.66113466765123E-16,1.,-5.66153840231349E-16));
#45364=DIRECTION('ref_axis',(0.957090014670973,-1.86337372849825E-16,0.289790793189011));
#45365=DIRECTION('center_axis',(3.66113466765123E-16,1.,-5.66153840231349E-16));
#45366=DIRECTION('ref_axis',(0.173514685168044,4.94039949369995E-16,0.98483128201283));
#45367=DIRECTION('center_axis',(-3.66113466765123E-16,-1.,5.66153840231349E-16));
#45368=DIRECTION('ref_axis',(-0.996957691137886,3.20870996777813E-16,-0.0779446090567869));
#45369=DIRECTION('center_axis',(3.66113466765123E-16,1.,-5.66153840231349E-16));
#45370=DIRECTION('ref_axis',(0.415642123266314,-6.67105086427771E-16,-0.909528243303456));
#45371=DIRECTION('center_axis',(3.66113466765123E-16,1.,-5.66153840231349E-16));
#45372=DIRECTION('ref_axis',(0.990639916096657,-2.85405978900105E-16,0.136501123204203));
#45373=DIRECTION('center_axis',(3.66113466765123E-16,1.,-5.66153840231349E-16));
#45374=DIRECTION('ref_axis',(0.325439986219075,4.16185990930063E-16,0.945562697746547));
#45375=DIRECTION('center_axis',(-3.66113466765123E-16,-1.,5.66153840231349E-16));
#45376=DIRECTION('ref_axis',(-0.996957691137886,3.20870996777813E-16,-0.0779446090567869));
#45377=DIRECTION('center_axis',(3.66113466765123E-16,1.,-5.66153840231349E-16));
#45378=DIRECTION('ref_axis',(0.268243314830189,-6.43612468217339E-16,-0.963351194554152));
#45379=DIRECTION('center_axis',(3.66113466765123E-16,1.,-5.66153840231349E-16));
#45380=DIRECTION('ref_axis',(0.999796975042654,-3.77446942541727E-16,-0.0201496574551476));
#45381=DIRECTION('center_axis',(3.66113466765123E-16,1.,-5.66153840231349E-16));
#45382=DIRECTION('ref_axis',(0.469351874736002,3.28084152151318E-16,0.883011221719068));
#45383=DIRECTION('center_axis',(-3.66113466765123E-16,-1.,5.66153840231349E-16));
#45384=DIRECTION('ref_axis',(-0.996957691137886,3.20870996777813E-16,-0.0779446090567869));
#45385=DIRECTION('center_axis',(3.66113466765123E-16,1.,-5.66153840231349E-16));
#45386=DIRECTION('ref_axis',(0.114239465734422,-6.04271975012079E-16,-0.993453242215613));
#45387=DIRECTION('center_axis',(3.66113466765123E-16,1.,-5.66153840231349E-16));
#45388=DIRECTION('ref_axis',(0.984335714327177,-4.60193909783388E-16,-0.176304286675074));
#45389=DIRECTION('center_axis',(3.66113466765123E-16,1.,-5.66153840231349E-16));
#45390=DIRECTION('ref_axis',(0.601706762407361,2.31903792697734E-16,0.798717078866636));
#45391=DIRECTION('center_axis',(-3.66113466765123E-16,-1.,5.66153840231349E-16));
#45392=DIRECTION('ref_axis',(-0.996957691137886,3.20870996777813E-16,-0.0779446090567869));
#45393=DIRECTION('center_axis',(3.66113466765123E-16,1.,-5.66153840231349E-16));
#45394=DIRECTION('ref_axis',(-0.0425773381467764,-5.50052300318313E-16,
-0.999093173971444));
#45395=DIRECTION('center_axis',(3.66113466765123E-16,1.,-5.66153840231349E-16));
#45396=DIRECTION('ref_axis',(0.944636841502024,-5.31609375670159E-16,-0.328117719236679));
#45397=DIRECTION('center_axis',(3.66113466765123E-16,1.,-5.66153840231349E-16));
#45398=DIRECTION('ref_axis',(0.719245632637998,1.30013192223369E-16,0.694755870742498));
#45399=DIRECTION('center_axis',(-3.66113466765123E-16,-1.,5.66153840231349E-16));
#45400=DIRECTION('ref_axis',(-0.996957691137886,3.20870996777813E-16,-0.0779446090567869));
#45401=DIRECTION('center_axis',(3.66113466765123E-16,1.,-5.66153840231349E-16));
#45402=DIRECTION('ref_axis',(-0.198345746656716,-4.82288512471788E-16,-0.980132115983957));
#45403=DIRECTION('center_axis',(3.66113466765123E-16,1.,-5.66153840231349E-16));
#45404=DIRECTION('ref_axis',(0.881677874569156,-5.89934854417565E-16,-0.471851804590399));
#45405=DIRECTION('center_axis',(3.66113466765123E-16,1.,-5.66153840231349E-16));
#45406=DIRECTION('ref_axis',(0.819074288353686,2.49212354674179E-17,0.573687467318141));
#45407=DIRECTION('center_axis',(-3.66113466765123E-16,-1.,5.66153840231349E-16));
#45408=DIRECTION('ref_axis',(-0.996957691137886,3.20870996777813E-16,-0.0779446090567869));
#45409=DIRECTION('center_axis',(3.66113466765123E-16,1.,-5.66153840231349E-16));
#45410=DIRECTION('ref_axis',(-0.349230224612176,-4.02649180824402E-16,-0.937036952428947));
#45411=DIRECTION('center_axis',(3.66113466765123E-16,1.,-5.66153840231349E-16));
#45412=DIRECTION('ref_axis',(0.797009072243291,-6.33734179167679E-16,-0.603967332528746));
#45413=DIRECTION('center_axis',(3.66113466765123E-16,1.,-5.66153840231349E-16));
#45414=DIRECTION('ref_axis',(0.898734616738394,-8.07843648145798E-17,0.438492974488865));
#45415=DIRECTION('center_axis',(-3.66113466765123E-16,-1.,5.66153840231349E-16));
#45416=DIRECTION('ref_axis',(-0.996957691137886,3.20870996777813E-16,-0.0779446090567869));
#45417=DIRECTION('center_axis',(3.66113466765123E-16,1.,-5.66153840231349E-16));
#45418=DIRECTION('ref_axis',(-0.491515495409017,-3.13095290029103E-16,-0.870868829257787));
#45419=DIRECTION('center_axis',(3.66113466765123E-16,1.,-5.66153840231349E-16));
#45420=DIRECTION('ref_axis',(0.692715261437337,-6.61928865183528E-16,-0.721211180287579));
#45421=DIRECTION('center_axis',(3.66113466765123E-16,1.,-5.66153840231349E-16));
#45422=DIRECTION('ref_axis',(0.956265116129817,-1.84500785926907E-16,0.292501329352925));
#45423=DIRECTION('center_axis',(-3.66113466765123E-16,-1.,5.66153840231349E-16));
#45424=DIRECTION('ref_axis',(-0.996957691137886,3.20870996777813E-16,-0.0779446090567869));
#45425=DIRECTION('center_axis',(3.66113466765123E-16,1.,-5.66153840231349E-16));
#45426=DIRECTION('ref_axis',(-0.621698023462484,-2.15831954089593E-16,-0.78325702526236));
#45427=DIRECTION('center_axis',(3.66113466765123E-16,1.,-5.66153840231349E-16));
#45428=DIRECTION('ref_axis',(0.571364501904649,-6.73824665722604E-16,-0.820696415225053));
#45429=DIRECTION('center_axis',(3.66113466765123E-16,1.,-5.66153840231349E-16));
#45430=DIRECTION('ref_axis',(0.990249194700156,-2.83674185366711E-16,0.139307330732061));
#45431=DIRECTION('center_axis',(-3.66113466765123E-16,-1.,5.66153840231349E-16));
#45432=DIRECTION('ref_axis',(-0.996957691137886,3.20870996777813E-16,-0.0779446090567869));
#45433=DIRECTION('center_axis',(3.66113466765123E-16,1.,-5.66153840231349E-16));
#45434=DIRECTION('ref_axis',(-0.736572282880858,-1.1325411913521E-16,-0.676358833823941));
#45435=DIRECTION('center_axis',(3.66113466765123E-16,1.,-5.66153840231349E-16));
#45436=DIRECTION('ref_axis',(0.435944852085004,-6.69128666695736E-16,-0.899973380684442));
#45437=DIRECTION('center_axis',(3.66113466765123E-16,1.,-5.66153840231349E-16));
#45438=DIRECTION('ref_axis',(0.999850051648321,-3.75862584902141E-16,-0.0173168767059515));
#45439=DIRECTION('center_axis',(-3.66113466765123E-16,-1.,5.66153840231349E-16));
#45440=DIRECTION('ref_axis',(-0.996957691137886,3.20870996777813E-16,-0.0779446090567869));
#45441=DIRECTION('center_axis',(3.66113466765123E-16,1.,-5.66153840231349E-16));
#45442=DIRECTION('ref_axis',(-0.833309688151449,-7.88759189884587E-18,-0.552806443190503));
#45443=DIRECTION('center_axis',(3.66113466765123E-16,1.,-5.66153840231349E-16));
#45444=DIRECTION('ref_axis',(0.289790793189011,-6.47956499184093E-16,-0.957090014670973));
#45445=DIRECTION('center_axis',(3.66113466765123E-16,1.,-5.66153840231349E-16));
#45446=DIRECTION('ref_axis',(0.98483128201283,-4.5879600018088E-16,-0.173514685168044));
#45447=DIRECTION('center_axis',(-3.66113466765123E-16,-1.,5.66153840231349E-16));
#45448=DIRECTION('ref_axis',(-0.996957691137886,3.20870996777813E-16,-0.0779446090567869));
#45449=DIRECTION('center_axis',(3.66113466765123E-16,1.,-5.66153840231349E-16));
#45450=DIRECTION('ref_axis',(-0.909528243303456,9.76731540274849E-17,-0.415642123266314));
#45451=DIRECTION('center_axis',(3.66113466765123E-16,1.,-5.66153840231349E-16));
#45452=DIRECTION('ref_axis',(0.136501123204203,-6.10829492218208E-16,-0.990639916096657));
#45453=DIRECTION('center_axis',(3.66113466765123E-16,1.,-5.66153840231349E-16));
#45454=DIRECTION('ref_axis',(0.945562697746547,-5.30432335278537E-16,-0.325439986219075));
#45455=DIRECTION('center_axis',(-3.66113466765123E-16,-1.,5.66153840231349E-16));
#45456=DIRECTION('ref_axis',(-0.996957691137886,3.20870996777813E-16,-0.0779446090567869));
#45457=DIRECTION('center_axis',(3.66113466765123E-16,1.,-5.66153840231349E-16));
#45458=DIRECTION('ref_axis',(-0.963351194554152,2.00828862743045E-16,-0.268243314830189));
#45459=DIRECTION('center_axis',(3.66113466765123E-16,1.,-5.66153840231349E-16));
#45460=DIRECTION('ref_axis',(-0.0201496574551477,-5.58661835927051E-16,
-0.999796975042654));
#45461=DIRECTION('center_axis',(3.66113466765123E-16,1.,-5.66153840231349E-16));
#45462=DIRECTION('ref_axis',(0.883011221719068,-5.89007665877645E-16,-0.469351874736002));
#45463=DIRECTION('center_axis',(-3.66113466765123E-16,-1.,5.66153840231349E-16));
#45464=DIRECTION('ref_axis',(-0.996957691137886,3.20870996777813E-16,-0.0779446090567869));
#45465=DIRECTION('center_axis',(0.0779446090567869,-5.92967996423326E-16,
-0.996957691137886));
#45466=DIRECTION('ref_axis',(0.996957691137886,-3.20870996777813E-16,0.0779446090567869));
#45467=DIRECTION('',(-0.996957691137886,3.20870996777813E-16,-0.0779446090567869));
#45468=DIRECTION('',(-3.66113466765123E-16,-1.,5.66153840231349E-16));
#45469=DIRECTION('',(-3.66113466765123E-16,-1.,5.66153840231349E-16));
#45470=DIRECTION('center_axis',(-0.996957691137886,3.20870996777813E-16,
-0.0779446090567869));
#45471=DIRECTION('ref_axis',(0.0779446090567869,-5.92967996423326E-16,-0.996957691137886));
#45472=DIRECTION('',(-0.0779446090567869,5.92967996423326E-16,0.996957691137886));
#45473=DIRECTION('',(3.66113466765123E-16,1.,-5.66153840231349E-16));
#45474=DIRECTION('center_axis',(-3.66113466765123E-16,-1.,5.66153840231349E-16));
#45475=DIRECTION('ref_axis',(-0.0779446090567859,5.92967996423326E-16,0.996957691137886));
#45476=DIRECTION('center_axis',(3.66113466765123E-16,1.,-5.66153840231349E-16));
#45477=DIRECTION('ref_axis',(-0.996957691137886,3.20870996777813E-16,-0.0779446090567869));
#45478=DIRECTION('',(-3.66113466765123E-16,-1.,5.66153840231349E-16));
#45479=DIRECTION('center_axis',(0.996957691137886,-3.20870996777813E-16,
0.0779446090567869));
#45480=DIRECTION('ref_axis',(-0.0779446090567869,5.92967996423326E-16,0.996957691137886));
#45481=DIRECTION('',(0.0779446090567869,-5.92967996423326E-16,-0.996957691137886));
#45482=DIRECTION('center_axis',(3.66113466765123E-16,1.,-5.66153840231349E-16));
#45483=DIRECTION('ref_axis',(-0.176304286675074,-4.92738071143036E-16,-0.984335714327177));
#45484=DIRECTION('',(3.66113466765123E-16,1.,-5.66153840231349E-16));
#45485=DIRECTION('center_axis',(-3.66113466765123E-16,-1.,5.66153840231349E-16));
#45486=DIRECTION('ref_axis',(-0.176304286675074,-4.92738071143036E-16,-0.984335714327177));
#45487=DIRECTION('',(3.66113466765123E-16,1.,-5.66153840231349E-16));
#45488=DIRECTION('center_axis',(3.66113466765123E-16,1.,-5.66153840231349E-16));
#45489=DIRECTION('ref_axis',(0.798717078866636,-6.33079672938476E-16,-0.601706762407361));
#45490=DIRECTION('center_axis',(-3.66113466765123E-16,-1.,5.66153840231349E-16));
#45491=DIRECTION('ref_axis',(0.798717078866636,-6.33079672938476E-16,-0.601706762407361));
#45492=DIRECTION('',(-3.66113466765123E-16,-1.,5.66153840231349E-16));
#45493=DIRECTION('center_axis',(3.66113466765123E-16,1.,-5.66153840231349E-16));
#45494=DIRECTION('ref_axis',(-0.993453242215613,2.99039498345089E-16,-0.114239465734422));
#45495=DIRECTION('',(3.66113466765123E-16,1.,-5.66153840231349E-16));
#45496=DIRECTION('center_axis',(-3.66113466765123E-16,-1.,5.66153840231349E-16));
#45497=DIRECTION('ref_axis',(-0.993453242215613,2.99039498345089E-16,-0.114239465734422));
#45498=DIRECTION('center_axis',(3.66113466765123E-16,1.,-5.66153840231349E-16));
#45499=DIRECTION('ref_axis',(-0.328117719236679,-4.14681459743577E-16,-0.944636841502024));
#45500=DIRECTION('',(3.66113466765123E-16,1.,-5.66153840231349E-16));
#45501=DIRECTION('center_axis',(-3.66113466765123E-16,-1.,5.66153840231349E-16));
#45502=DIRECTION('ref_axis',(-0.328117719236679,-4.14681459743577E-16,-0.944636841502024));
#45503=DIRECTION('',(3.66113466765123E-16,1.,-5.66153840231349E-16));
#45504=DIRECTION('center_axis',(3.66113466765123E-16,1.,-5.66153840231349E-16));
#45505=DIRECTION('ref_axis',(0.694755870742498,-6.61563157380586E-16,-0.719245632637998));
#45506=DIRECTION('center_axis',(-3.66113466765123E-16,-1.,5.66153840231349E-16));
#45507=DIRECTION('ref_axis',(0.694755870742498,-6.61563157380586E-16,-0.719245632637998));
#45508=DIRECTION('',(-3.66113466765123E-16,-1.,5.66153840231349E-16));
#45509=DIRECTION('center_axis',(3.66113466765123E-16,1.,-5.66153840231349E-16));
#45510=DIRECTION('ref_axis',(-0.999093173971444,3.89886789042682E-16,0.0425773381467764));
#45511=DIRECTION('',(3.66113466765123E-16,1.,-5.66153840231349E-16));
#45512=DIRECTION('center_axis',(-3.66113466765123E-16,-1.,5.66153840231349E-16));
#45513=DIRECTION('ref_axis',(-0.999093173971444,3.89886789042682E-16,0.0425773381467764));
#45514=DIRECTION('center_axis',(3.66113466765123E-16,1.,-5.66153840231349E-16));
#45515=DIRECTION('ref_axis',(-0.471851804590399,-3.26414014556371E-16,-0.881677874569156));
#45516=DIRECTION('',(3.66113466765123E-16,1.,-5.66153840231349E-16));
#45517=DIRECTION('center_axis',(-3.66113466765123E-16,-1.,5.66153840231349E-16));
#45518=DIRECTION('ref_axis',(-0.471851804590399,-3.26414014556371E-16,-0.881677874569156));
#45519=DIRECTION('',(3.66113466765123E-16,1.,-5.66153840231349E-16));
#45520=DIRECTION('center_axis',(3.66113466765123E-16,1.,-5.66153840231349E-16));
#45521=DIRECTION('ref_axis',(0.573687467318141,-6.73756761285746E-16,-0.819074288353686));
#45522=DIRECTION('center_axis',(-3.66113466765123E-16,-1.,5.66153840231349E-16));
#45523=DIRECTION('ref_axis',(0.573687467318141,-6.73756761285746E-16,-0.819074288353686));
#45524=DIRECTION('',(-3.66113466765123E-16,-1.,5.66153840231349E-16));
#45525=DIRECTION('center_axis',(3.66113466765123E-16,1.,-5.66153840231349E-16));
#45526=DIRECTION('ref_axis',(-0.980132115983957,4.71133773033976E-16,0.198345746656716));
#45527=DIRECTION('',(3.66113466765123E-16,1.,-5.66153840231349E-16));
#45528=DIRECTION('center_axis',(-3.66113466765123E-16,-1.,5.66153840231349E-16));
#45529=DIRECTION('ref_axis',(-0.980132115983957,4.71133773033976E-16,0.198345746656716));
#45530=DIRECTION('center_axis',(3.66113466765123E-16,1.,-5.66153840231349E-16));
#45531=DIRECTION('ref_axis',(-0.603967332528746,-2.30109173024781E-16,-0.797009072243291));
#45532=DIRECTION('',(3.66113466765123E-16,1.,-5.66153840231349E-16));
#45533=DIRECTION('center_axis',(-3.66113466765123E-16,-1.,5.66153840231349E-16));
#45534=DIRECTION('ref_axis',(-0.603967332528746,-2.30109173024781E-16,-0.797009072243291));
#45535=DIRECTION('',(3.66113466765123E-16,1.,-5.66153840231349E-16));
#45536=DIRECTION('center_axis',(3.66113466765123E-16,1.,-5.66153840231349E-16));
#45537=DIRECTION('ref_axis',(0.438492974488865,-6.6936023765756E-16,-0.898734616738394));
#45538=DIRECTION('center_axis',(-3.66113466765123E-16,-1.,5.66153840231349E-16));
#45539=DIRECTION('ref_axis',(0.438492974488865,-6.6936023765756E-16,-0.898734616738394));
#45540=DIRECTION('',(-3.66113466765123E-16,-1.,5.66153840231349E-16));
#45541=DIRECTION('center_axis',(3.66113466765123E-16,1.,-5.66153840231349E-16));
#45542=DIRECTION('ref_axis',(-0.937036952428947,5.40779879929828E-16,0.349230224612176));
#45543=DIRECTION('',(3.66113466765123E-16,1.,-5.66153840231349E-16));
#45544=DIRECTION('center_axis',(-3.66113466765123E-16,-1.,5.66153840231349E-16));
#45545=DIRECTION('ref_axis',(-0.937036952428947,5.40779879929828E-16,0.349230224612176));
#45546=DIRECTION('center_axis',(3.66113466765123E-16,1.,-5.66153840231349E-16));
#45547=DIRECTION('ref_axis',(-0.721211180287579,-1.28138279964759E-16,-0.692715261437336));
#45548=DIRECTION('',(3.66113466765123E-16,1.,-5.66153840231349E-16));
#45549=DIRECTION('center_axis',(-3.66113466765123E-16,-1.,5.66153840231349E-16));
#45550=DIRECTION('ref_axis',(-0.721211180287579,-1.28138279964759E-16,-0.692715261437336));
#45551=DIRECTION('',(3.66113466765123E-16,1.,-5.66153840231349E-16));
#45552=DIRECTION('center_axis',(3.66113466765123E-16,1.,-5.66153840231349E-16));
#45553=DIRECTION('ref_axis',(0.292501329352925,-6.48481843498979E-16,-0.956265116129817));
#45554=DIRECTION('center_axis',(-3.66113466765123E-16,-1.,5.66153840231349E-16));
#45555=DIRECTION('ref_axis',(0.292501329352925,-6.48481843498979E-16,-0.956265116129817));
#45556=DIRECTION('',(-3.66113466765123E-16,-1.,5.66153840231349E-16));
#45557=DIRECTION('center_axis',(3.66113466765123E-16,1.,-5.66153840231349E-16));
#45558=DIRECTION('ref_axis',(-0.870868829257786,5.97110191436282E-16,0.491515495409018));
#45559=DIRECTION('',(3.66113466765123E-16,1.,-5.66153840231349E-16));
#45560=DIRECTION('center_axis',(-3.66113466765123E-16,-1.,5.66153840231349E-16));
#45561=DIRECTION('ref_axis',(-0.870868829257786,5.97110191436282E-16,0.491515495409018));
#45562=DIRECTION('center_axis',(3.66113466765123E-16,1.,-5.66153840231349E-16));
#45563=DIRECTION('ref_axis',(-0.820696415225053,-2.30121971854362E-17,-0.571364501904649));
#45564=DIRECTION('',(3.66113466765123E-16,1.,-5.66153840231349E-16));
#45565=DIRECTION('center_axis',(-3.66113466765123E-16,-1.,5.66153840231349E-16));
#45566=DIRECTION('ref_axis',(-0.820696415225053,-2.30121971854362E-17,-0.571364501904649));
#45567=DIRECTION('',(3.66113466765123E-16,1.,-5.66153840231349E-16));
#45568=DIRECTION('center_axis',(3.66113466765123E-16,1.,-5.66153840231349E-16));
#45569=DIRECTION('ref_axis',(0.139307330732061,-6.11635674165605E-16,-0.990249194700156));
#45570=DIRECTION('center_axis',(-3.66113466765123E-16,-1.,5.66153840231349E-16));
#45571=DIRECTION('ref_axis',(0.139307330732061,-6.11635674165605E-16,-0.990249194700156));
#45572=DIRECTION('',(-3.66113466765123E-16,-1.,5.66153840231349E-16));
#45573=DIRECTION('center_axis',(3.66113466765123E-16,1.,-5.66153840231349E-16));
#45574=DIRECTION('ref_axis',(-0.78325702526236,6.38737668334465E-16,0.621698023462484));
#45575=DIRECTION('',(3.66113466765123E-16,1.,-5.66153840231349E-16));
#45576=DIRECTION('center_axis',(-3.66113466765123E-16,-1.,5.66153840231349E-16));
#45577=DIRECTION('ref_axis',(-0.78325702526236,6.38737668334465E-16,0.621698023462484));
#45578=DIRECTION('center_axis',(3.66113466765123E-16,1.,-5.66153840231349E-16));
#45579=DIRECTION('ref_axis',(-0.899973380684442,8.26805222616965E-17,-0.435944852085004));
#45580=DIRECTION('',(3.66113466765123E-16,1.,-5.66153840231349E-16));
#45581=DIRECTION('center_axis',(-3.66113466765123E-16,-1.,5.66153840231349E-16));
#45582=DIRECTION('ref_axis',(-0.899973380684442,8.26805222616965E-17,-0.435944852085004));
#45583=DIRECTION('',(3.66113466765123E-16,1.,-5.66153840231349E-16));
#45584=DIRECTION('center_axis',(3.66113466765123E-16,1.,-5.66153840231349E-16));
#45585=DIRECTION('ref_axis',(-0.0173168767059515,-5.5972900463185E-16,-0.999850051648321));
#45586=DIRECTION('center_axis',(-3.66113466765123E-16,-1.,5.66153840231349E-16));
#45587=DIRECTION('ref_axis',(-0.0173168767059515,-5.5972900463185E-16,-0.999850051648321));
#45588=DIRECTION('',(-3.66113466765123E-16,-1.,5.66153840231349E-16));
#45589=DIRECTION('center_axis',(3.66113466765123E-16,1.,-5.66153840231349E-16));
#45590=DIRECTION('ref_axis',(-0.676358833823941,6.64637303989468E-16,0.736572282880858));
#45591=DIRECTION('',(3.66113466765123E-16,1.,-5.66153840231349E-16));
#45592=DIRECTION('center_axis',(-3.66113466765123E-16,-1.,5.66153840231349E-16));
#45593=DIRECTION('ref_axis',(-0.676358833823941,6.64637303989468E-16,0.736572282880858));
#45594=DIRECTION('center_axis',(3.66113466765123E-16,1.,-5.66153840231349E-16));
#45595=DIRECTION('ref_axis',(-0.957090014670973,1.86337372849825E-16,-0.289790793189011));
#45596=DIRECTION('',(3.66113466765123E-16,1.,-5.66153840231349E-16));
#45597=DIRECTION('center_axis',(-3.66113466765123E-16,-1.,5.66153840231349E-16));
#45598=DIRECTION('ref_axis',(-0.957090014670973,1.86337372849825E-16,-0.289790793189011));
#45599=DIRECTION('',(3.66113466765123E-16,1.,-5.66153840231349E-16));
#45600=DIRECTION('center_axis',(3.66113466765123E-16,1.,-5.66153840231349E-16));
#45601=DIRECTION('ref_axis',(-0.173514685168044,-4.94039949369995E-16,-0.98483128201283));
#45602=DIRECTION('center_axis',(-3.66113466765123E-16,-1.,5.66153840231349E-16));
#45603=DIRECTION('ref_axis',(-0.173514685168044,-4.94039949369995E-16,-0.98483128201283));
#45604=DIRECTION('',(-3.66113466765123E-16,-1.,5.66153840231349E-16));
#45605=DIRECTION('center_axis',(3.66113466765123E-16,1.,-5.66153840231349E-16));
#45606=DIRECTION('ref_axis',(-0.552806443190503,6.74171363415503E-16,0.833309688151449));
#45607=DIRECTION('',(3.66113466765123E-16,1.,-5.66153840231349E-16));
#45608=DIRECTION('center_axis',(-3.66113466765123E-16,-1.,5.66153840231349E-16));
#45609=DIRECTION('ref_axis',(-0.552806443190503,6.74171363415503E-16,0.833309688151449));
#45610=DIRECTION('center_axis',(3.66113466765123E-16,1.,-5.66153840231349E-16));
#45611=DIRECTION('ref_axis',(-0.990639916096657,2.85405978900106E-16,-0.136501123204203));
#45612=DIRECTION('',(3.66113466765123E-16,1.,-5.66153840231349E-16));
#45613=DIRECTION('center_axis',(-3.66113466765123E-16,-1.,5.66153840231349E-16));
#45614=DIRECTION('ref_axis',(-0.990639916096657,2.85405978900106E-16,-0.136501123204203));
#45615=DIRECTION('',(3.66113466765123E-16,1.,-5.66153840231349E-16));
#45616=DIRECTION('center_axis',(3.66113466765123E-16,1.,-5.66153840231349E-16));
#45617=DIRECTION('ref_axis',(-0.325439986219075,-4.16185990930063E-16,-0.945562697746547));
#45618=DIRECTION('center_axis',(-3.66113466765123E-16,-1.,5.66153840231349E-16));
#45619=DIRECTION('ref_axis',(-0.325439986219075,-4.16185990930063E-16,-0.945562697746547));
#45620=DIRECTION('',(-3.66113466765123E-16,-1.,5.66153840231349E-16));
#45621=DIRECTION('center_axis',(3.66113466765123E-16,1.,-5.66153840231349E-16));
#45622=DIRECTION('ref_axis',(-0.415642123266314,6.67105086427771E-16,0.909528243303456));
#45623=DIRECTION('',(3.66113466765123E-16,1.,-5.66153840231349E-16));
#45624=DIRECTION('center_axis',(-3.66113466765123E-16,-1.,5.66153840231349E-16));
#45625=DIRECTION('ref_axis',(-0.415642123266314,6.67105086427771E-16,0.909528243303456));
#45626=DIRECTION('center_axis',(3.66113466765123E-16,1.,-5.66153840231349E-16));
#45627=DIRECTION('ref_axis',(-0.999796975042654,3.77446942541727E-16,0.0201496574551479));
#45628=DIRECTION('',(3.66113466765123E-16,1.,-5.66153840231349E-16));
#45629=DIRECTION('center_axis',(-3.66113466765123E-16,-1.,5.66153840231349E-16));
#45630=DIRECTION('ref_axis',(-0.999796975042654,3.77446942541727E-16,0.0201496574551479));
#45631=DIRECTION('',(3.66113466765123E-16,1.,-5.66153840231349E-16));
#45632=DIRECTION('center_axis',(3.66113466765123E-16,1.,-5.66153840231349E-16));
#45633=DIRECTION('ref_axis',(-0.469351874736002,-3.28084152151318E-16,-0.883011221719068));
#45634=DIRECTION('center_axis',(-3.66113466765123E-16,-1.,5.66153840231349E-16));
#45635=DIRECTION('ref_axis',(-0.469351874736002,-3.28084152151318E-16,-0.883011221719068));
#45636=DIRECTION('',(-3.66113466765123E-16,-1.,5.66153840231349E-16));
#45637=DIRECTION('center_axis',(3.66113466765123E-16,1.,-5.66153840231349E-16));
#45638=DIRECTION('ref_axis',(-0.268243314830189,6.43612468217339E-16,0.963351194554152));
#45639=DIRECTION('',(3.66113466765123E-16,1.,-5.66153840231349E-16));
#45640=DIRECTION('center_axis',(-3.66113466765123E-16,-1.,5.66153840231349E-16));
#45641=DIRECTION('ref_axis',(-0.268243314830189,6.43612468217339E-16,0.963351194554152));
#45642=DIRECTION('center_axis',(3.66113466765123E-16,1.,-5.66153840231349E-16));
#45643=DIRECTION('ref_axis',(-0.984335714327177,4.60193909783388E-16,0.176304286675074));
#45644=DIRECTION('',(3.66113466765123E-16,1.,-5.66153840231349E-16));
#45645=DIRECTION('center_axis',(-3.66113466765123E-16,-1.,5.66153840231349E-16));
#45646=DIRECTION('ref_axis',(-0.984335714327177,4.60193909783388E-16,0.176304286675074));
#45647=DIRECTION('',(3.66113466765123E-16,1.,-5.66153840231349E-16));
#45648=DIRECTION('center_axis',(3.66113466765123E-16,1.,-5.66153840231349E-16));
#45649=DIRECTION('ref_axis',(-0.601706762407361,-2.31903792697734E-16,-0.798717078866636));
#45650=DIRECTION('center_axis',(-3.66113466765123E-16,-1.,5.66153840231349E-16));
#45651=DIRECTION('ref_axis',(-0.601706762407361,-2.31903792697734E-16,-0.798717078866636));
#45652=DIRECTION('',(-3.66113466765123E-16,-1.,5.66153840231349E-16));
#45653=DIRECTION('center_axis',(3.66113466765123E-16,1.,-5.66153840231349E-16));
#45654=DIRECTION('ref_axis',(-0.114239465734422,6.04271975012079E-16,0.993453242215613));
#45655=DIRECTION('',(3.66113466765123E-16,1.,-5.66153840231349E-16));
#45656=DIRECTION('center_axis',(-3.66113466765123E-16,-1.,5.66153840231349E-16));
#45657=DIRECTION('ref_axis',(-0.114239465734422,6.04271975012079E-16,0.993453242215613));
#45658=DIRECTION('center_axis',(3.66113466765123E-16,1.,-5.66153840231349E-16));
#45659=DIRECTION('ref_axis',(-0.944636841502024,5.31609375670159E-16,0.328117719236679));
#45660=DIRECTION('',(3.66113466765123E-16,1.,-5.66153840231349E-16));
#45661=DIRECTION('center_axis',(-3.66113466765123E-16,-1.,5.66153840231349E-16));
#45662=DIRECTION('ref_axis',(-0.944636841502024,5.31609375670159E-16,0.328117719236679));
#45663=DIRECTION('',(3.66113466765123E-16,1.,-5.66153840231349E-16));
#45664=DIRECTION('center_axis',(3.66113466765123E-16,1.,-5.66153840231349E-16));
#45665=DIRECTION('ref_axis',(-0.719245632637998,-1.30013192223369E-16,-0.694755870742498));
#45666=DIRECTION('center_axis',(-3.66113466765123E-16,-1.,5.66153840231349E-16));
#45667=DIRECTION('ref_axis',(-0.719245632637998,-1.30013192223369E-16,-0.694755870742498));
#45668=DIRECTION('',(-3.66113466765123E-16,-1.,5.66153840231349E-16));
#45669=DIRECTION('center_axis',(3.66113466765123E-16,1.,-5.66153840231349E-16));
#45670=DIRECTION('ref_axis',(0.0425773381467764,5.50052300318313E-16,0.999093173971444));
#45671=DIRECTION('',(3.66113466765123E-16,1.,-5.66153840231349E-16));
#45672=DIRECTION('center_axis',(-3.66113466765123E-16,-1.,5.66153840231349E-16));
#45673=DIRECTION('ref_axis',(0.0425773381467764,5.50052300318313E-16,0.999093173971444));
#45674=DIRECTION('center_axis',(3.66113466765123E-16,1.,-5.66153840231349E-16));
#45675=DIRECTION('ref_axis',(-0.881677874569156,5.89934854417565E-16,0.471851804590399));
#45676=DIRECTION('',(3.66113466765123E-16,1.,-5.66153840231349E-16));
#45677=DIRECTION('center_axis',(-3.66113466765123E-16,-1.,5.66153840231349E-16));
#45678=DIRECTION('ref_axis',(-0.881677874569156,5.89934854417565E-16,0.471851804590399));
#45679=DIRECTION('',(3.66113466765123E-16,1.,-5.66153840231349E-16));
#45680=DIRECTION('center_axis',(3.66113466765123E-16,1.,-5.66153840231349E-16));
#45681=DIRECTION('ref_axis',(-0.819074288353686,-2.49212354674179E-17,-0.573687467318141));
#45682=DIRECTION('center_axis',(-3.66113466765123E-16,-1.,5.66153840231349E-16));
#45683=DIRECTION('ref_axis',(-0.819074288353686,-2.49212354674179E-17,-0.573687467318141));
#45684=DIRECTION('',(-3.66113466765123E-16,-1.,5.66153840231349E-16));
#45685=DIRECTION('center_axis',(3.66113466765123E-16,1.,-5.66153840231349E-16));
#45686=DIRECTION('ref_axis',(0.198345746656716,4.82288512471788E-16,0.980132115983957));
#45687=DIRECTION('',(3.66113466765123E-16,1.,-5.66153840231349E-16));
#45688=DIRECTION('center_axis',(-3.66113466765123E-16,-1.,5.66153840231349E-16));
#45689=DIRECTION('ref_axis',(0.198345746656716,4.82288512471788E-16,0.980132115983957));
#45690=DIRECTION('center_axis',(3.66113466765123E-16,1.,-5.66153840231349E-16));
#45691=DIRECTION('ref_axis',(-0.797009072243291,6.33734179167679E-16,0.603967332528746));
#45692=DIRECTION('',(3.66113466765123E-16,1.,-5.66153840231349E-16));
#45693=DIRECTION('center_axis',(-3.66113466765123E-16,-1.,5.66153840231349E-16));
#45694=DIRECTION('ref_axis',(-0.797009072243291,6.33734179167679E-16,0.603967332528746));
#45695=DIRECTION('',(3.66113466765123E-16,1.,-5.66153840231349E-16));
#45696=DIRECTION('center_axis',(3.66113466765123E-16,1.,-5.66153840231349E-16));
#45697=DIRECTION('ref_axis',(-0.898734616738394,8.07843648145798E-17,-0.438492974488865));
#45698=DIRECTION('center_axis',(-3.66113466765123E-16,-1.,5.66153840231349E-16));
#45699=DIRECTION('ref_axis',(-0.898734616738394,8.07843648145798E-17,-0.438492974488865));
#45700=DIRECTION('',(-3.66113466765123E-16,-1.,5.66153840231349E-16));
#45701=DIRECTION('center_axis',(3.66113466765123E-16,1.,-5.66153840231349E-16));
#45702=DIRECTION('ref_axis',(0.349230224612176,4.02649180824402E-16,0.937036952428947));
#45703=DIRECTION('',(3.66113466765123E-16,1.,-5.66153840231349E-16));
#45704=DIRECTION('center_axis',(-3.66113466765123E-16,-1.,5.66153840231349E-16));
#45705=DIRECTION('ref_axis',(0.349230224612176,4.02649180824402E-16,0.937036952428947));
#45706=DIRECTION('center_axis',(3.66113466765123E-16,1.,-5.66153840231349E-16));
#45707=DIRECTION('ref_axis',(-0.692715261437337,6.61928865183528E-16,0.721211180287579));
#45708=DIRECTION('',(3.66113466765123E-16,1.,-5.66153840231349E-16));
#45709=DIRECTION('center_axis',(-3.66113466765123E-16,-1.,5.66153840231349E-16));
#45710=DIRECTION('ref_axis',(-0.692715261437337,6.61928865183528E-16,0.721211180287579));
#45711=DIRECTION('',(3.66113466765123E-16,1.,-5.66153840231349E-16));
#45712=DIRECTION('center_axis',(3.66113466765123E-16,1.,-5.66153840231349E-16));
#45713=DIRECTION('ref_axis',(-0.956265116129817,1.84500785926907E-16,-0.292501329352925));
#45714=DIRECTION('center_axis',(-3.66113466765123E-16,-1.,5.66153840231349E-16));
#45715=DIRECTION('ref_axis',(-0.956265116129817,1.84500785926907E-16,-0.292501329352925));
#45716=DIRECTION('',(-3.66113466765123E-16,-1.,5.66153840231349E-16));
#45717=DIRECTION('center_axis',(3.66113466765123E-16,1.,-5.66153840231349E-16));
#45718=DIRECTION('ref_axis',(0.491515495409017,3.13095290029103E-16,0.870868829257787));
#45719=DIRECTION('',(3.66113466765123E-16,1.,-5.66153840231349E-16));
#45720=DIRECTION('center_axis',(-3.66113466765123E-16,-1.,5.66153840231349E-16));
#45721=DIRECTION('ref_axis',(0.491515495409017,3.13095290029103E-16,0.870868829257787));
#45722=DIRECTION('center_axis',(3.66113466765123E-16,1.,-5.66153840231349E-16));
#45723=DIRECTION('ref_axis',(-0.571364501904649,6.73824665722604E-16,0.820696415225053));
#45724=DIRECTION('',(3.66113466765123E-16,1.,-5.66153840231349E-16));
#45725=DIRECTION('center_axis',(-3.66113466765123E-16,-1.,5.66153840231349E-16));
#45726=DIRECTION('ref_axis',(-0.571364501904649,6.73824665722604E-16,0.820696415225053));
#45727=DIRECTION('',(3.66113466765123E-16,1.,-5.66153840231349E-16));
#45728=DIRECTION('center_axis',(3.66113466765123E-16,1.,-5.66153840231349E-16));
#45729=DIRECTION('ref_axis',(-0.990249194700156,2.83674185366711E-16,-0.13930733073206));
#45730=DIRECTION('center_axis',(-3.66113466765123E-16,-1.,5.66153840231349E-16));
#45731=DIRECTION('ref_axis',(-0.990249194700156,2.83674185366711E-16,-0.13930733073206));
#45732=DIRECTION('',(-3.66113466765123E-16,-1.,5.66153840231349E-16));
#45733=DIRECTION('center_axis',(3.66113466765123E-16,1.,-5.66153840231349E-16));
#45734=DIRECTION('ref_axis',(0.621698023462484,2.15831954089593E-16,0.78325702526236));
#45735=DIRECTION('',(3.66113466765123E-16,1.,-5.66153840231349E-16));
#45736=DIRECTION('center_axis',(-3.66113466765123E-16,-1.,5.66153840231349E-16));
#45737=DIRECTION('ref_axis',(0.621698023462484,2.15831954089593E-16,0.78325702526236));
#45738=DIRECTION('center_axis',(3.66113466765123E-16,1.,-5.66153840231349E-16));
#45739=DIRECTION('ref_axis',(-0.435944852085004,6.69128666695736E-16,0.899973380684442));
#45740=DIRECTION('',(3.66113466765123E-16,1.,-5.66153840231349E-16));
#45741=DIRECTION('center_axis',(-3.66113466765123E-16,-1.,5.66153840231349E-16));
#45742=DIRECTION('ref_axis',(-0.435944852085004,6.69128666695736E-16,0.899973380684442));
#45743=DIRECTION('',(3.66113466765123E-16,1.,-5.66153840231349E-16));
#45744=DIRECTION('center_axis',(3.66113466765123E-16,1.,-5.66153840231349E-16));
#45745=DIRECTION('ref_axis',(-0.999850051648321,3.75862584902141E-16,0.0173168767059515));
#45746=DIRECTION('center_axis',(-3.66113466765123E-16,-1.,5.66153840231349E-16));
#45747=DIRECTION('ref_axis',(-0.999850051648321,3.75862584902141E-16,0.0173168767059515));
#45748=DIRECTION('',(-3.66113466765123E-16,-1.,5.66153840231349E-16));
#45749=DIRECTION('center_axis',(3.66113466765123E-16,1.,-5.66153840231349E-16));
#45750=DIRECTION('ref_axis',(0.736572282880858,1.1325411913521E-16,0.676358833823941));
#45751=DIRECTION('',(3.66113466765123E-16,1.,-5.66153840231349E-16));
#45752=DIRECTION('center_axis',(-3.66113466765123E-16,-1.,5.66153840231349E-16));
#45753=DIRECTION('ref_axis',(0.736572282880858,1.1325411913521E-16,0.676358833823941));
#45754=DIRECTION('center_axis',(3.66113466765123E-16,1.,-5.66153840231349E-16));
#45755=DIRECTION('ref_axis',(-0.289790793189011,6.47956499184093E-16,0.957090014670973));
#45756=DIRECTION('',(3.66113466765123E-16,1.,-5.66153840231349E-16));
#45757=DIRECTION('center_axis',(-3.66113466765123E-16,-1.,5.66153840231349E-16));
#45758=DIRECTION('ref_axis',(-0.289790793189011,6.47956499184093E-16,0.957090014670973));
#45759=DIRECTION('',(3.66113466765123E-16,1.,-5.66153840231349E-16));
#45760=DIRECTION('center_axis',(3.66113466765123E-16,1.,-5.66153840231349E-16));
#45761=DIRECTION('ref_axis',(-0.98483128201283,4.5879600018088E-16,0.173514685168044));
#45762=DIRECTION('center_axis',(-3.66113466765123E-16,-1.,5.66153840231349E-16));
#45763=DIRECTION('ref_axis',(-0.98483128201283,4.5879600018088E-16,0.173514685168044));
#45764=DIRECTION('',(-3.66113466765123E-16,-1.,5.66153840231349E-16));
#45765=DIRECTION('center_axis',(3.66113466765123E-16,1.,-5.66153840231349E-16));
#45766=DIRECTION('ref_axis',(0.833309688151449,7.88759189884587E-18,0.552806443190503));
#45767=DIRECTION('',(3.66113466765123E-16,1.,-5.66153840231349E-16));
#45768=DIRECTION('center_axis',(-3.66113466765123E-16,-1.,5.66153840231349E-16));
#45769=DIRECTION('ref_axis',(0.833309688151449,7.88759189884587E-18,0.552806443190503));
#45770=DIRECTION('center_axis',(3.66113466765123E-16,1.,-5.66153840231349E-16));
#45771=DIRECTION('ref_axis',(-0.136501123204203,6.10829492218208E-16,0.990639916096657));
#45772=DIRECTION('',(3.66113466765123E-16,1.,-5.66153840231349E-16));
#45773=DIRECTION('center_axis',(-3.66113466765123E-16,-1.,5.66153840231349E-16));
#45774=DIRECTION('ref_axis',(-0.136501123204203,6.10829492218208E-16,0.990639916096657));
#45775=DIRECTION('',(3.66113466765123E-16,1.,-5.66153840231349E-16));
#45776=DIRECTION('center_axis',(3.66113466765123E-16,1.,-5.66153840231349E-16));
#45777=DIRECTION('ref_axis',(-0.945562697746547,5.30432335278537E-16,0.325439986219075));
#45778=DIRECTION('center_axis',(-3.66113466765123E-16,-1.,5.66153840231349E-16));
#45779=DIRECTION('ref_axis',(-0.945562697746547,5.30432335278537E-16,0.325439986219075));
#45780=DIRECTION('',(-3.66113466765123E-16,-1.,5.66153840231349E-16));
#45781=DIRECTION('center_axis',(3.66113466765123E-16,1.,-5.66153840231349E-16));
#45782=DIRECTION('ref_axis',(0.909528243303456,-9.76731540274849E-17,0.415642123266314));
#45783=DIRECTION('',(3.66113466765123E-16,1.,-5.66153840231349E-16));
#45784=DIRECTION('center_axis',(-3.66113466765123E-16,-1.,5.66153840231349E-16));
#45785=DIRECTION('ref_axis',(0.909528243303456,-9.76731540274849E-17,0.415642123266314));
#45786=DIRECTION('center_axis',(3.66113466765123E-16,1.,-5.66153840231349E-16));
#45787=DIRECTION('ref_axis',(0.0201496574551478,5.58661835927051E-16,0.999796975042654));
#45788=DIRECTION('',(3.66113466765123E-16,1.,-5.66153840231349E-16));
#45789=DIRECTION('center_axis',(-3.66113466765123E-16,-1.,5.66153840231349E-16));
#45790=DIRECTION('ref_axis',(0.0201496574551478,5.58661835927051E-16,0.999796975042654));
#45791=DIRECTION('',(3.66113466765123E-16,1.,-5.66153840231349E-16));
#45792=DIRECTION('center_axis',(3.66113466765123E-16,1.,-5.66153840231349E-16));
#45793=DIRECTION('ref_axis',(-0.883011221719068,5.89007665877645E-16,0.469351874736002));
#45794=DIRECTION('center_axis',(-3.66113466765123E-16,-1.,5.66153840231349E-16));
#45795=DIRECTION('ref_axis',(-0.883011221719068,5.89007665877645E-16,0.469351874736002));
#45796=DIRECTION('',(-3.66113466765123E-16,-1.,5.66153840231349E-16));
#45797=DIRECTION('center_axis',(3.66113466765123E-16,1.,-5.66153840231349E-16));
#45798=DIRECTION('ref_axis',(0.963351194554152,-2.00828862743045E-16,0.268243314830189));
#45799=DIRECTION('',(3.66113466765123E-16,1.,-5.66153840231349E-16));
#45800=DIRECTION('center_axis',(-3.66113466765123E-16,-1.,5.66153840231349E-16));
#45801=DIRECTION('ref_axis',(0.963351194554152,-2.00828862743045E-16,0.268243314830189));
#45802=DIRECTION('center_axis',(3.66113466765123E-16,1.,-5.66153840231349E-16));
#45803=DIRECTION('ref_axis',(0.176304286675074,4.92738071143036E-16,0.984335714327177));
#45804=DIRECTION('',(3.66113466765123E-16,1.,-5.66153840231349E-16));
#45805=DIRECTION('center_axis',(-3.66113466765123E-16,-1.,5.66153840231349E-16));
#45806=DIRECTION('ref_axis',(0.176304286675074,4.92738071143036E-16,0.984335714327177));
#45807=DIRECTION('',(3.66113466765123E-16,1.,-5.66153840231349E-16));
#45808=DIRECTION('center_axis',(3.66113466765123E-16,1.,-5.66153840231349E-16));
#45809=DIRECTION('ref_axis',(-0.798717078866636,6.33079672938476E-16,0.601706762407361));
#45810=DIRECTION('center_axis',(-3.66113466765123E-16,-1.,5.66153840231349E-16));
#45811=DIRECTION('ref_axis',(-0.798717078866636,6.33079672938476E-16,0.601706762407361));
#45812=DIRECTION('',(-3.66113466765123E-16,-1.,5.66153840231349E-16));
#45813=DIRECTION('center_axis',(3.66113466765123E-16,1.,-5.66153840231349E-16));
#45814=DIRECTION('ref_axis',(0.993453242215613,-2.99039498345089E-16,0.114239465734422));
#45815=DIRECTION('',(3.66113466765123E-16,1.,-5.66153840231349E-16));
#45816=DIRECTION('center_axis',(-3.66113466765123E-16,-1.,5.66153840231349E-16));
#45817=DIRECTION('ref_axis',(0.993453242215613,-2.99039498345089E-16,0.114239465734422));
#45818=DIRECTION('center_axis',(3.66113466765123E-16,1.,-5.66153840231349E-16));
#45819=DIRECTION('ref_axis',(0.328117719236679,4.14681459743577E-16,0.944636841502024));
#45820=DIRECTION('',(3.66113466765123E-16,1.,-5.66153840231349E-16));
#45821=DIRECTION('center_axis',(-3.66113466765123E-16,-1.,5.66153840231349E-16));
#45822=DIRECTION('ref_axis',(0.328117719236679,4.14681459743577E-16,0.944636841502024));
#45823=DIRECTION('',(3.66113466765123E-16,1.,-5.66153840231349E-16));
#45824=DIRECTION('center_axis',(3.66113466765123E-16,1.,-5.66153840231349E-16));
#45825=DIRECTION('ref_axis',(-0.694755870742498,6.61563157380586E-16,0.719245632637998));
#45826=DIRECTION('center_axis',(-3.66113466765123E-16,-1.,5.66153840231349E-16));
#45827=DIRECTION('ref_axis',(-0.694755870742498,6.61563157380586E-16,0.719245632637998));
#45828=DIRECTION('',(-3.66113466765123E-16,-1.,5.66153840231349E-16));
#45829=DIRECTION('center_axis',(3.66113466765123E-16,1.,-5.66153840231349E-16));
#45830=DIRECTION('ref_axis',(0.999093173971444,-3.89886789042682E-16,-0.0425773381467764));
#45831=DIRECTION('',(3.66113466765123E-16,1.,-5.66153840231349E-16));
#45832=DIRECTION('center_axis',(-3.66113466765123E-16,-1.,5.66153840231349E-16));
#45833=DIRECTION('ref_axis',(0.999093173971444,-3.89886789042682E-16,-0.0425773381467764));
#45834=DIRECTION('center_axis',(3.66113466765123E-16,1.,-5.66153840231349E-16));
#45835=DIRECTION('ref_axis',(0.471851804590399,3.26414014556371E-16,0.881677874569156));
#45836=DIRECTION('',(3.66113466765123E-16,1.,-5.66153840231349E-16));
#45837=DIRECTION('center_axis',(-3.66113466765123E-16,-1.,5.66153840231349E-16));
#45838=DIRECTION('ref_axis',(0.471851804590399,3.26414014556371E-16,0.881677874569156));
#45839=DIRECTION('',(3.66113466765123E-16,1.,-5.66153840231349E-16));
#45840=DIRECTION('center_axis',(3.66113466765123E-16,1.,-5.66153840231349E-16));
#45841=DIRECTION('ref_axis',(-0.573687467318141,6.73756761285746E-16,0.819074288353686));
#45842=DIRECTION('center_axis',(-3.66113466765123E-16,-1.,5.66153840231349E-16));
#45843=DIRECTION('ref_axis',(-0.573687467318141,6.73756761285746E-16,0.819074288353686));
#45844=DIRECTION('',(-3.66113466765123E-16,-1.,5.66153840231349E-16));
#45845=DIRECTION('center_axis',(3.66113466765123E-16,1.,-5.66153840231349E-16));
#45846=DIRECTION('ref_axis',(0.980132115983957,-4.71133773033976E-16,-0.198345746656716));
#45847=DIRECTION('',(3.66113466765123E-16,1.,-5.66153840231349E-16));
#45848=DIRECTION('center_axis',(-3.66113466765123E-16,-1.,5.66153840231349E-16));
#45849=DIRECTION('ref_axis',(0.980132115983957,-4.71133773033976E-16,-0.198345746656716));
#45850=DIRECTION('center_axis',(3.66113466765123E-16,1.,-5.66153840231349E-16));
#45851=DIRECTION('ref_axis',(0.603967332528746,2.30109173024781E-16,0.797009072243291));
#45852=DIRECTION('',(3.66113466765123E-16,1.,-5.66153840231349E-16));
#45853=DIRECTION('center_axis',(-3.66113466765123E-16,-1.,5.66153840231349E-16));
#45854=DIRECTION('ref_axis',(0.603967332528746,2.30109173024781E-16,0.797009072243291));
#45855=DIRECTION('',(3.66113466765123E-16,1.,-5.66153840231349E-16));
#45856=DIRECTION('center_axis',(3.66113466765123E-16,1.,-5.66153840231349E-16));
#45857=DIRECTION('ref_axis',(-0.438492974488865,6.6936023765756E-16,0.898734616738394));
#45858=DIRECTION('center_axis',(-3.66113466765123E-16,-1.,5.66153840231349E-16));
#45859=DIRECTION('ref_axis',(-0.438492974488865,6.6936023765756E-16,0.898734616738394));
#45860=DIRECTION('',(-3.66113466765123E-16,-1.,5.66153840231349E-16));
#45861=DIRECTION('center_axis',(3.66113466765123E-16,1.,-5.66153840231349E-16));
#45862=DIRECTION('ref_axis',(0.937036952428947,-5.40779879929828E-16,-0.349230224612176));
#45863=DIRECTION('',(3.66113466765123E-16,1.,-5.66153840231349E-16));
#45864=DIRECTION('center_axis',(-3.66113466765123E-16,-1.,5.66153840231349E-16));
#45865=DIRECTION('ref_axis',(0.937036952428947,-5.40779879929828E-16,-0.349230224612176));
#45866=DIRECTION('center_axis',(3.66113466765123E-16,1.,-5.66153840231349E-16));
#45867=DIRECTION('ref_axis',(0.721211180287579,1.2813827996476E-16,0.692715261437337));
#45868=DIRECTION('',(3.66113466765123E-16,1.,-5.66153840231349E-16));
#45869=DIRECTION('center_axis',(-3.66113466765123E-16,-1.,5.66153840231349E-16));
#45870=DIRECTION('ref_axis',(0.721211180287579,1.2813827996476E-16,0.692715261437337));
#45871=DIRECTION('',(3.66113466765123E-16,1.,-5.66153840231349E-16));
#45872=DIRECTION('center_axis',(3.66113466765123E-16,1.,-5.66153840231349E-16));
#45873=DIRECTION('ref_axis',(-0.292501329352925,6.48481843498979E-16,0.956265116129817));
#45874=DIRECTION('center_axis',(-3.66113466765123E-16,-1.,5.66153840231349E-16));
#45875=DIRECTION('ref_axis',(-0.292501329352925,6.48481843498979E-16,0.956265116129817));
#45876=DIRECTION('',(-3.66113466765123E-16,-1.,5.66153840231349E-16));
#45877=DIRECTION('center_axis',(3.66113466765123E-16,1.,-5.66153840231349E-16));
#45878=DIRECTION('ref_axis',(0.870868829257786,-5.97110191436282E-16,-0.491515495409018));
#45879=DIRECTION('',(3.66113466765123E-16,1.,-5.66153840231349E-16));
#45880=DIRECTION('center_axis',(-3.66113466765123E-16,-1.,5.66153840231349E-16));
#45881=DIRECTION('ref_axis',(0.870868829257786,-5.97110191436282E-16,-0.491515495409018));
#45882=DIRECTION('center_axis',(3.66113466765123E-16,1.,-5.66153840231349E-16));
#45883=DIRECTION('ref_axis',(0.820696415225053,2.30121971854362E-17,0.571364501904649));
#45884=DIRECTION('',(3.66113466765123E-16,1.,-5.66153840231349E-16));
#45885=DIRECTION('center_axis',(-3.66113466765123E-16,-1.,5.66153840231349E-16));
#45886=DIRECTION('ref_axis',(0.820696415225053,2.30121971854362E-17,0.571364501904649));
#45887=DIRECTION('',(3.66113466765123E-16,1.,-5.66153840231349E-16));
#45888=DIRECTION('center_axis',(3.66113466765123E-16,1.,-5.66153840231349E-16));
#45889=DIRECTION('ref_axis',(-0.13930733073206,6.11635674165605E-16,0.990249194700156));
#45890=DIRECTION('center_axis',(-3.66113466765123E-16,-1.,5.66153840231349E-16));
#45891=DIRECTION('ref_axis',(-0.13930733073206,6.11635674165605E-16,0.990249194700156));
#45892=DIRECTION('',(-3.66113466765123E-16,-1.,5.66153840231349E-16));
#45893=DIRECTION('center_axis',(3.66113466765123E-16,1.,-5.66153840231349E-16));
#45894=DIRECTION('ref_axis',(0.78325702526236,-6.38737668334465E-16,-0.621698023462484));
#45895=DIRECTION('',(3.66113466765123E-16,1.,-5.66153840231349E-16));
#45896=DIRECTION('center_axis',(-3.66113466765123E-16,-1.,5.66153840231349E-16));
#45897=DIRECTION('ref_axis',(0.78325702526236,-6.38737668334465E-16,-0.621698023462484));
#45898=DIRECTION('center_axis',(3.66113466765123E-16,1.,-5.66153840231349E-16));
#45899=DIRECTION('ref_axis',(0.899973380684442,-8.26805222616965E-17,0.435944852085004));
#45900=DIRECTION('',(3.66113466765123E-16,1.,-5.66153840231349E-16));
#45901=DIRECTION('center_axis',(-3.66113466765123E-16,-1.,5.66153840231349E-16));
#45902=DIRECTION('ref_axis',(0.899973380684442,-8.26805222616965E-17,0.435944852085004));
#45903=DIRECTION('',(3.66113466765123E-16,1.,-5.66153840231349E-16));
#45904=DIRECTION('center_axis',(3.66113466765123E-16,1.,-5.66153840231349E-16));
#45905=DIRECTION('ref_axis',(0.0173168767059515,5.5972900463185E-16,0.999850051648321));
#45906=DIRECTION('center_axis',(-3.66113466765123E-16,-1.,5.66153840231349E-16));
#45907=DIRECTION('ref_axis',(0.0173168767059515,5.5972900463185E-16,0.999850051648321));
#45908=DIRECTION('',(-3.66113466765123E-16,-1.,5.66153840231349E-16));
#45909=DIRECTION('center_axis',(3.66113466765123E-16,1.,-5.66153840231349E-16));
#45910=DIRECTION('ref_axis',(0.676358833823941,-6.64637303989468E-16,-0.736572282880858));
#45911=DIRECTION('',(3.66113466765123E-16,1.,-5.66153840231349E-16));
#45912=DIRECTION('center_axis',(-3.66113466765123E-16,-1.,5.66153840231349E-16));
#45913=DIRECTION('ref_axis',(0.676358833823941,-6.64637303989468E-16,-0.736572282880858));
#45914=DIRECTION('center_axis',(3.66113466765123E-16,1.,-5.66153840231349E-16));
#45915=DIRECTION('ref_axis',(0.957090014670973,-1.86337372849825E-16,0.289790793189011));
#45916=DIRECTION('',(3.66113466765123E-16,1.,-5.66153840231349E-16));
#45917=DIRECTION('center_axis',(-3.66113466765123E-16,-1.,5.66153840231349E-16));
#45918=DIRECTION('ref_axis',(0.957090014670973,-1.86337372849825E-16,0.289790793189011));
#45919=DIRECTION('',(3.66113466765123E-16,1.,-5.66153840231349E-16));
#45920=DIRECTION('center_axis',(3.66113466765123E-16,1.,-5.66153840231349E-16));
#45921=DIRECTION('ref_axis',(0.173514685168044,4.94039949369995E-16,0.98483128201283));
#45922=DIRECTION('center_axis',(-3.66113466765123E-16,-1.,5.66153840231349E-16));
#45923=DIRECTION('ref_axis',(0.173514685168044,4.94039949369995E-16,0.98483128201283));
#45924=DIRECTION('',(-3.66113466765123E-16,-1.,5.66153840231349E-16));
#45925=DIRECTION('center_axis',(3.66113466765123E-16,1.,-5.66153840231349E-16));
#45926=DIRECTION('ref_axis',(0.552806443190503,-6.74171363415503E-16,-0.833309688151449));
#45927=DIRECTION('',(3.66113466765123E-16,1.,-5.66153840231349E-16));
#45928=DIRECTION('center_axis',(-3.66113466765123E-16,-1.,5.66153840231349E-16));
#45929=DIRECTION('ref_axis',(0.552806443190503,-6.74171363415503E-16,-0.833309688151449));
#45930=DIRECTION('center_axis',(3.66113466765123E-16,1.,-5.66153840231349E-16));
#45931=DIRECTION('ref_axis',(0.990639916096657,-2.85405978900105E-16,0.136501123204203));
#45932=DIRECTION('',(3.66113466765123E-16,1.,-5.66153840231349E-16));
#45933=DIRECTION('center_axis',(-3.66113466765123E-16,-1.,5.66153840231349E-16));
#45934=DIRECTION('ref_axis',(0.990639916096657,-2.85405978900105E-16,0.136501123204203));
#45935=DIRECTION('',(3.66113466765123E-16,1.,-5.66153840231349E-16));
#45936=DIRECTION('center_axis',(3.66113466765123E-16,1.,-5.66153840231349E-16));
#45937=DIRECTION('ref_axis',(0.325439986219075,4.16185990930063E-16,0.945562697746547));
#45938=DIRECTION('center_axis',(-3.66113466765123E-16,-1.,5.66153840231349E-16));
#45939=DIRECTION('ref_axis',(0.325439986219075,4.16185990930063E-16,0.945562697746547));
#45940=DIRECTION('',(-3.66113466765123E-16,-1.,5.66153840231349E-16));
#45941=DIRECTION('center_axis',(3.66113466765123E-16,1.,-5.66153840231349E-16));
#45942=DIRECTION('ref_axis',(0.415642123266314,-6.67105086427771E-16,-0.909528243303456));
#45943=DIRECTION('',(3.66113466765123E-16,1.,-5.66153840231349E-16));
#45944=DIRECTION('center_axis',(-3.66113466765123E-16,-1.,5.66153840231349E-16));
#45945=DIRECTION('ref_axis',(0.415642123266314,-6.67105086427771E-16,-0.909528243303456));
#45946=DIRECTION('center_axis',(3.66113466765123E-16,1.,-5.66153840231349E-16));
#45947=DIRECTION('ref_axis',(0.999796975042654,-3.77446942541727E-16,-0.0201496574551476));
#45948=DIRECTION('',(3.66113466765123E-16,1.,-5.66153840231349E-16));
#45949=DIRECTION('center_axis',(-3.66113466765123E-16,-1.,5.66153840231349E-16));
#45950=DIRECTION('ref_axis',(0.999796975042654,-3.77446942541727E-16,-0.0201496574551476));
#45951=DIRECTION('',(3.66113466765123E-16,1.,-5.66153840231349E-16));
#45952=DIRECTION('center_axis',(3.66113466765123E-16,1.,-5.66153840231349E-16));
#45953=DIRECTION('ref_axis',(0.469351874736002,3.28084152151318E-16,0.883011221719068));
#45954=DIRECTION('center_axis',(-3.66113466765123E-16,-1.,5.66153840231349E-16));
#45955=DIRECTION('ref_axis',(0.469351874736002,3.28084152151318E-16,0.883011221719068));
#45956=DIRECTION('',(-3.66113466765123E-16,-1.,5.66153840231349E-16));
#45957=DIRECTION('center_axis',(3.66113466765123E-16,1.,-5.66153840231349E-16));
#45958=DIRECTION('ref_axis',(0.268243314830189,-6.43612468217339E-16,-0.963351194554152));
#45959=DIRECTION('',(3.66113466765123E-16,1.,-5.66153840231349E-16));
#45960=DIRECTION('center_axis',(-3.66113466765123E-16,-1.,5.66153840231349E-16));
#45961=DIRECTION('ref_axis',(0.268243314830189,-6.43612468217339E-16,-0.963351194554152));
#45962=DIRECTION('center_axis',(3.66113466765123E-16,1.,-5.66153840231349E-16));
#45963=DIRECTION('ref_axis',(0.984335714327177,-4.60193909783388E-16,-0.176304286675074));
#45964=DIRECTION('',(3.66113466765123E-16,1.,-5.66153840231349E-16));
#45965=DIRECTION('center_axis',(-3.66113466765123E-16,-1.,5.66153840231349E-16));
#45966=DIRECTION('ref_axis',(0.984335714327177,-4.60193909783388E-16,-0.176304286675074));
#45967=DIRECTION('',(3.66113466765123E-16,1.,-5.66153840231349E-16));
#45968=DIRECTION('center_axis',(3.66113466765123E-16,1.,-5.66153840231349E-16));
#45969=DIRECTION('ref_axis',(0.601706762407361,2.31903792697734E-16,0.798717078866636));
#45970=DIRECTION('center_axis',(-3.66113466765123E-16,-1.,5.66153840231349E-16));
#45971=DIRECTION('ref_axis',(0.601706762407361,2.31903792697734E-16,0.798717078866636));
#45972=DIRECTION('',(-3.66113466765123E-16,-1.,5.66153840231349E-16));
#45973=DIRECTION('center_axis',(3.66113466765123E-16,1.,-5.66153840231349E-16));
#45974=DIRECTION('ref_axis',(0.114239465734422,-6.04271975012079E-16,-0.993453242215613));
#45975=DIRECTION('',(3.66113466765123E-16,1.,-5.66153840231349E-16));
#45976=DIRECTION('center_axis',(-3.66113466765123E-16,-1.,5.66153840231349E-16));
#45977=DIRECTION('ref_axis',(0.114239465734422,-6.04271975012079E-16,-0.993453242215613));
#45978=DIRECTION('center_axis',(3.66113466765123E-16,1.,-5.66153840231349E-16));
#45979=DIRECTION('ref_axis',(0.944636841502024,-5.31609375670159E-16,-0.328117719236679));
#45980=DIRECTION('',(3.66113466765123E-16,1.,-5.66153840231349E-16));
#45981=DIRECTION('center_axis',(-3.66113466765123E-16,-1.,5.66153840231349E-16));
#45982=DIRECTION('ref_axis',(0.944636841502024,-5.31609375670159E-16,-0.328117719236679));
#45983=DIRECTION('',(3.66113466765123E-16,1.,-5.66153840231349E-16));
#45984=DIRECTION('center_axis',(3.66113466765123E-16,1.,-5.66153840231349E-16));
#45985=DIRECTION('ref_axis',(0.719245632637998,1.30013192223369E-16,0.694755870742498));
#45986=DIRECTION('center_axis',(-3.66113466765123E-16,-1.,5.66153840231349E-16));
#45987=DIRECTION('ref_axis',(0.719245632637998,1.30013192223369E-16,0.694755870742498));
#45988=DIRECTION('',(-3.66113466765123E-16,-1.,5.66153840231349E-16));
#45989=DIRECTION('center_axis',(3.66113466765123E-16,1.,-5.66153840231349E-16));
#45990=DIRECTION('ref_axis',(-0.0425773381467764,-5.50052300318313E-16,
-0.999093173971444));
#45991=DIRECTION('',(3.66113466765123E-16,1.,-5.66153840231349E-16));
#45992=DIRECTION('center_axis',(-3.66113466765123E-16,-1.,5.66153840231349E-16));
#45993=DIRECTION('ref_axis',(-0.0425773381467764,-5.50052300318313E-16,
-0.999093173971444));
#45994=DIRECTION('center_axis',(3.66113466765123E-16,1.,-5.66153840231349E-16));
#45995=DIRECTION('ref_axis',(0.881677874569156,-5.89934854417565E-16,-0.471851804590399));
#45996=DIRECTION('',(3.66113466765123E-16,1.,-5.66153840231349E-16));
#45997=DIRECTION('center_axis',(-3.66113466765123E-16,-1.,5.66153840231349E-16));
#45998=DIRECTION('ref_axis',(0.881677874569156,-5.89934854417565E-16,-0.471851804590399));
#45999=DIRECTION('',(3.66113466765123E-16,1.,-5.66153840231349E-16));
#46000=DIRECTION('center_axis',(3.66113466765123E-16,1.,-5.66153840231349E-16));
#46001=DIRECTION('ref_axis',(0.819074288353686,2.49212354674179E-17,0.573687467318141));
#46002=DIRECTION('center_axis',(-3.66113466765123E-16,-1.,5.66153840231349E-16));
#46003=DIRECTION('ref_axis',(0.819074288353686,2.49212354674179E-17,0.573687467318141));
#46004=DIRECTION('',(-3.66113466765123E-16,-1.,5.66153840231349E-16));
#46005=DIRECTION('center_axis',(3.66113466765123E-16,1.,-5.66153840231349E-16));
#46006=DIRECTION('ref_axis',(-0.198345746656716,-4.82288512471788E-16,-0.980132115983957));
#46007=DIRECTION('',(3.66113466765123E-16,1.,-5.66153840231349E-16));
#46008=DIRECTION('center_axis',(-3.66113466765123E-16,-1.,5.66153840231349E-16));
#46009=DIRECTION('ref_axis',(-0.198345746656716,-4.82288512471788E-16,-0.980132115983957));
#46010=DIRECTION('center_axis',(3.66113466765123E-16,1.,-5.66153840231349E-16));
#46011=DIRECTION('ref_axis',(0.797009072243291,-6.33734179167679E-16,-0.603967332528746));
#46012=DIRECTION('',(3.66113466765123E-16,1.,-5.66153840231349E-16));
#46013=DIRECTION('center_axis',(-3.66113466765123E-16,-1.,5.66153840231349E-16));
#46014=DIRECTION('ref_axis',(0.797009072243291,-6.33734179167679E-16,-0.603967332528746));
#46015=DIRECTION('',(3.66113466765123E-16,1.,-5.66153840231349E-16));
#46016=DIRECTION('center_axis',(3.66113466765123E-16,1.,-5.66153840231349E-16));
#46017=DIRECTION('ref_axis',(0.898734616738394,-8.07843648145798E-17,0.438492974488865));
#46018=DIRECTION('center_axis',(-3.66113466765123E-16,-1.,5.66153840231349E-16));
#46019=DIRECTION('ref_axis',(0.898734616738394,-8.07843648145798E-17,0.438492974488865));
#46020=DIRECTION('',(-3.66113466765123E-16,-1.,5.66153840231349E-16));
#46021=DIRECTION('center_axis',(3.66113466765123E-16,1.,-5.66153840231349E-16));
#46022=DIRECTION('ref_axis',(-0.349230224612176,-4.02649180824402E-16,-0.937036952428947));
#46023=DIRECTION('',(3.66113466765123E-16,1.,-5.66153840231349E-16));
#46024=DIRECTION('center_axis',(-3.66113466765123E-16,-1.,5.66153840231349E-16));
#46025=DIRECTION('ref_axis',(-0.349230224612176,-4.02649180824402E-16,-0.937036952428947));
#46026=DIRECTION('center_axis',(3.66113466765123E-16,1.,-5.66153840231349E-16));
#46027=DIRECTION('ref_axis',(0.692715261437337,-6.61928865183528E-16,-0.721211180287579));
#46028=DIRECTION('',(3.66113466765123E-16,1.,-5.66153840231349E-16));
#46029=DIRECTION('center_axis',(-3.66113466765123E-16,-1.,5.66153840231349E-16));
#46030=DIRECTION('ref_axis',(0.692715261437337,-6.61928865183528E-16,-0.721211180287579));
#46031=DIRECTION('',(3.66113466765123E-16,1.,-5.66153840231349E-16));
#46032=DIRECTION('center_axis',(3.66113466765123E-16,1.,-5.66153840231349E-16));
#46033=DIRECTION('ref_axis',(0.956265116129817,-1.84500785926907E-16,0.292501329352925));
#46034=DIRECTION('center_axis',(-3.66113466765123E-16,-1.,5.66153840231349E-16));
#46035=DIRECTION('ref_axis',(0.956265116129817,-1.84500785926907E-16,0.292501329352925));
#46036=DIRECTION('',(-3.66113466765123E-16,-1.,5.66153840231349E-16));
#46037=DIRECTION('center_axis',(3.66113466765123E-16,1.,-5.66153840231349E-16));
#46038=DIRECTION('ref_axis',(-0.491515495409017,-3.13095290029103E-16,-0.870868829257787));
#46039=DIRECTION('',(3.66113466765123E-16,1.,-5.66153840231349E-16));
#46040=DIRECTION('center_axis',(-3.66113466765123E-16,-1.,5.66153840231349E-16));
#46041=DIRECTION('ref_axis',(-0.491515495409017,-3.13095290029103E-16,-0.870868829257787));
#46042=DIRECTION('center_axis',(3.66113466765123E-16,1.,-5.66153840231349E-16));
#46043=DIRECTION('ref_axis',(0.571364501904649,-6.73824665722604E-16,-0.820696415225053));
#46044=DIRECTION('',(3.66113466765123E-16,1.,-5.66153840231349E-16));
#46045=DIRECTION('center_axis',(-3.66113466765123E-16,-1.,5.66153840231349E-16));
#46046=DIRECTION('ref_axis',(0.571364501904649,-6.73824665722604E-16,-0.820696415225053));
#46047=DIRECTION('',(3.66113466765123E-16,1.,-5.66153840231349E-16));
#46048=DIRECTION('center_axis',(3.66113466765123E-16,1.,-5.66153840231349E-16));
#46049=DIRECTION('ref_axis',(0.990249194700156,-2.83674185366711E-16,0.139307330732061));
#46050=DIRECTION('center_axis',(-3.66113466765123E-16,-1.,5.66153840231349E-16));
#46051=DIRECTION('ref_axis',(0.990249194700156,-2.83674185366711E-16,0.139307330732061));
#46052=DIRECTION('',(-3.66113466765123E-16,-1.,5.66153840231349E-16));
#46053=DIRECTION('center_axis',(3.66113466765123E-16,1.,-5.66153840231349E-16));
#46054=DIRECTION('ref_axis',(-0.621698023462484,-2.15831954089593E-16,-0.78325702526236));
#46055=DIRECTION('',(3.66113466765123E-16,1.,-5.66153840231349E-16));
#46056=DIRECTION('center_axis',(-3.66113466765123E-16,-1.,5.66153840231349E-16));
#46057=DIRECTION('ref_axis',(-0.621698023462484,-2.15831954089593E-16,-0.78325702526236));
#46058=DIRECTION('center_axis',(3.66113466765123E-16,1.,-5.66153840231349E-16));
#46059=DIRECTION('ref_axis',(0.435944852085004,-6.69128666695736E-16,-0.899973380684442));
#46060=DIRECTION('',(3.66113466765123E-16,1.,-5.66153840231349E-16));
#46061=DIRECTION('center_axis',(-3.66113466765123E-16,-1.,5.66153840231349E-16));
#46062=DIRECTION('ref_axis',(0.435944852085004,-6.69128666695736E-16,-0.899973380684442));
#46063=DIRECTION('',(3.66113466765123E-16,1.,-5.66153840231349E-16));
#46064=DIRECTION('center_axis',(3.66113466765123E-16,1.,-5.66153840231349E-16));
#46065=DIRECTION('ref_axis',(0.999850051648321,-3.75862584902141E-16,-0.0173168767059515));
#46066=DIRECTION('center_axis',(-3.66113466765123E-16,-1.,5.66153840231349E-16));
#46067=DIRECTION('ref_axis',(0.999850051648321,-3.75862584902141E-16,-0.0173168767059515));
#46068=DIRECTION('',(-3.66113466765123E-16,-1.,5.66153840231349E-16));
#46069=DIRECTION('center_axis',(3.66113466765123E-16,1.,-5.66153840231349E-16));
#46070=DIRECTION('ref_axis',(-0.736572282880858,-1.1325411913521E-16,-0.676358833823941));
#46071=DIRECTION('',(3.66113466765123E-16,1.,-5.66153840231349E-16));
#46072=DIRECTION('center_axis',(-3.66113466765123E-16,-1.,5.66153840231349E-16));
#46073=DIRECTION('ref_axis',(-0.736572282880858,-1.1325411913521E-16,-0.676358833823941));
#46074=DIRECTION('center_axis',(3.66113466765123E-16,1.,-5.66153840231349E-16));
#46075=DIRECTION('ref_axis',(0.289790793189011,-6.47956499184093E-16,-0.957090014670973));
#46076=DIRECTION('',(3.66113466765123E-16,1.,-5.66153840231349E-16));
#46077=DIRECTION('center_axis',(-3.66113466765123E-16,-1.,5.66153840231349E-16));
#46078=DIRECTION('ref_axis',(0.289790793189011,-6.47956499184093E-16,-0.957090014670973));
#46079=DIRECTION('',(3.66113466765123E-16,1.,-5.66153840231349E-16));
#46080=DIRECTION('center_axis',(3.66113466765123E-16,1.,-5.66153840231349E-16));
#46081=DIRECTION('ref_axis',(0.98483128201283,-4.5879600018088E-16,-0.173514685168044));
#46082=DIRECTION('center_axis',(-3.66113466765123E-16,-1.,5.66153840231349E-16));
#46083=DIRECTION('ref_axis',(0.98483128201283,-4.5879600018088E-16,-0.173514685168044));
#46084=DIRECTION('',(-3.66113466765123E-16,-1.,5.66153840231349E-16));
#46085=DIRECTION('center_axis',(3.66113466765123E-16,1.,-5.66153840231349E-16));
#46086=DIRECTION('ref_axis',(-0.833309688151449,-7.88759189884587E-18,-0.552806443190503));
#46087=DIRECTION('',(3.66113466765123E-16,1.,-5.66153840231349E-16));
#46088=DIRECTION('center_axis',(-3.66113466765123E-16,-1.,5.66153840231349E-16));
#46089=DIRECTION('ref_axis',(-0.833309688151449,-7.88759189884587E-18,-0.552806443190503));
#46090=DIRECTION('center_axis',(3.66113466765123E-16,1.,-5.66153840231349E-16));
#46091=DIRECTION('ref_axis',(0.136501123204203,-6.10829492218208E-16,-0.990639916096657));
#46092=DIRECTION('',(3.66113466765123E-16,1.,-5.66153840231349E-16));
#46093=DIRECTION('center_axis',(-3.66113466765123E-16,-1.,5.66153840231349E-16));
#46094=DIRECTION('ref_axis',(0.136501123204203,-6.10829492218208E-16,-0.990639916096657));
#46095=DIRECTION('',(3.66113466765123E-16,1.,-5.66153840231349E-16));
#46096=DIRECTION('center_axis',(3.66113466765123E-16,1.,-5.66153840231349E-16));
#46097=DIRECTION('ref_axis',(0.945562697746547,-5.30432335278537E-16,-0.325439986219075));
#46098=DIRECTION('center_axis',(-3.66113466765123E-16,-1.,5.66153840231349E-16));
#46099=DIRECTION('ref_axis',(0.945562697746547,-5.30432335278537E-16,-0.325439986219075));
#46100=DIRECTION('',(-3.66113466765123E-16,-1.,5.66153840231349E-16));
#46101=DIRECTION('center_axis',(3.66113466765123E-16,1.,-5.66153840231349E-16));
#46102=DIRECTION('ref_axis',(-0.909528243303456,9.76731540274849E-17,-0.415642123266314));
#46103=DIRECTION('',(3.66113466765123E-16,1.,-5.66153840231349E-16));
#46104=DIRECTION('center_axis',(-3.66113466765123E-16,-1.,5.66153840231349E-16));
#46105=DIRECTION('ref_axis',(-0.909528243303456,9.76731540274849E-17,-0.415642123266314));
#46106=DIRECTION('center_axis',(3.66113466765123E-16,1.,-5.66153840231349E-16));
#46107=DIRECTION('ref_axis',(-0.996957691137886,3.20870996777813E-16,-0.0779446090567869));
#46108=DIRECTION('center_axis',(-3.66113466765123E-16,-1.,5.66153840231349E-16));
#46109=DIRECTION('ref_axis',(-0.996957691137886,3.20870996777813E-16,-0.0779446090567869));
#46110=DIRECTION('',(3.66113466765123E-16,1.,-5.66153840231349E-16));
#46111=DIRECTION('center_axis',(3.66113466765123E-16,1.,-5.66153840231349E-16));
#46112=DIRECTION('ref_axis',(-0.996957691137886,3.20870996777813E-16,-0.0779446090567869));
#46113=DIRECTION('center_axis',(-3.66113466765123E-16,-1.,5.66153840231349E-16));
#46114=DIRECTION('ref_axis',(-0.996957691137886,3.20870996777813E-16,-0.0779446090567869));
#46115=DIRECTION('center_axis',(3.66113466765123E-16,1.,-5.66153840231349E-16));
#46116=DIRECTION('ref_axis',(-0.996957691137886,3.20870996777813E-16,-0.0779446090567869));
#46117=DIRECTION('center_axis',(-3.66113466765123E-16,-1.,5.66153840231349E-16));
#46118=DIRECTION('ref_axis',(-0.996957691137886,3.20870996777813E-16,-0.0779446090567869));
#46119=DIRECTION('center_axis',(3.66113466765123E-16,1.,-5.66153840231349E-16));
#46120=DIRECTION('ref_axis',(-0.996957691137886,3.20870996777813E-16,-0.0779446090567869));
#46121=DIRECTION('center_axis',(-3.66113466765123E-16,-1.,5.66153840231349E-16));
#46122=DIRECTION('ref_axis',(-0.996957691137886,3.20870996777813E-16,-0.0779446090567869));
#46123=DIRECTION('center_axis',(3.66113466765123E-16,1.,-5.66153840231349E-16));
#46124=DIRECTION('ref_axis',(-0.996957691137886,3.20870996777813E-16,-0.0779446090567869));
#46125=DIRECTION('center_axis',(-3.66113466765123E-16,-1.,5.66153840231349E-16));
#46126=DIRECTION('ref_axis',(-0.996957691137886,3.20870996777813E-16,-0.0779446090567869));
#46127=DIRECTION('center_axis',(3.66113466765123E-16,1.,-5.66153840231349E-16));
#46128=DIRECTION('ref_axis',(-0.996957691137886,3.20870996777813E-16,-0.0779446090567869));
#46129=DIRECTION('center_axis',(-3.66113466765123E-16,-1.,5.66153840231349E-16));
#46130=DIRECTION('ref_axis',(-0.996957691137886,3.20870996777813E-16,-0.0779446090567869));
#46131=DIRECTION('center_axis',(3.66113466765123E-16,1.,-5.66153840231349E-16));
#46132=DIRECTION('ref_axis',(-0.996957691137886,3.20870996777813E-16,-0.0779446090567869));
#46133=DIRECTION('center_axis',(-3.66113466765123E-16,-1.,5.66153840231349E-16));
#46134=DIRECTION('ref_axis',(-0.996957691137886,3.20870996777813E-16,-0.0779446090567869));
#46135=DIRECTION('center_axis',(3.66113466765123E-16,1.,-5.66153840231349E-16));
#46136=DIRECTION('ref_axis',(-0.996957691137886,3.20870996777813E-16,-0.0779446090567869));
#46137=DIRECTION('center_axis',(-3.66113466765123E-16,-1.,5.66153840231349E-16));
#46138=DIRECTION('ref_axis',(-0.996957691137886,3.20870996777813E-16,-0.0779446090567869));
#46139=DIRECTION('center_axis',(3.66113466765123E-16,1.,-5.66153840231349E-16));
#46140=DIRECTION('ref_axis',(-0.996957691137886,3.20870996777813E-16,-0.0779446090567869));
#46141=DIRECTION('center_axis',(-3.66113466765123E-16,-1.,5.66153840231349E-16));
#46142=DIRECTION('ref_axis',(-0.996957691137886,3.20870996777813E-16,-0.0779446090567869));
#46143=DIRECTION('center_axis',(3.66113466765123E-16,1.,-5.66153840231349E-16));
#46144=DIRECTION('ref_axis',(-0.996957691137886,3.20870996777813E-16,-0.0779446090567869));
#46145=DIRECTION('center_axis',(-3.66113466765123E-16,-1.,5.66153840231349E-16));
#46146=DIRECTION('ref_axis',(-0.996957691137886,3.20870996777813E-16,-0.0779446090567869));
#46147=DIRECTION('center_axis',(3.66113466765123E-16,1.,-5.66153840231349E-16));
#46148=DIRECTION('ref_axis',(0.996957691137886,-3.20870996777813E-16,0.0779446090567866));
#46149=DIRECTION('center_axis',(-3.66113466765123E-16,-1.,5.66153840231349E-16));
#46150=DIRECTION('ref_axis',(-0.996957691137886,3.20870996777813E-16,-0.0779446090567869));
#46151=DIRECTION('center_axis',(3.66113466765123E-16,1.,-5.66153840231349E-16));
#46152=DIRECTION('ref_axis',(-0.996957691137886,3.20870996777813E-16,-0.0779446090567869));
#46153=DIRECTION('center_axis',(-3.66113466765123E-16,-1.,5.66153840231349E-16));
#46154=DIRECTION('ref_axis',(-0.996957691137886,3.20870996777813E-16,-0.0779446090567869));
#46155=DIRECTION('center_axis',(3.66113466765123E-16,1.,-5.66153840231349E-16));
#46156=DIRECTION('ref_axis',(-0.996957691137886,3.20870996777813E-16,-0.0779446090567869));
#46157=DIRECTION('center_axis',(-3.66113466765123E-16,-1.,5.66153840231349E-16));
#46158=DIRECTION('ref_axis',(-0.996957691137886,3.20870996777813E-16,-0.0779446090567869));
#46159=DIRECTION('center_axis',(3.66113466765123E-16,1.,-5.66153840231349E-16));
#46160=DIRECTION('ref_axis',(-0.996957691137886,3.20870996777813E-16,-0.0779446090567869));
#46161=DIRECTION('center_axis',(-3.66113466765123E-16,-1.,5.66153840231349E-16));
#46162=DIRECTION('ref_axis',(-0.996957691137886,3.20870996777813E-16,-0.0779446090567869));
#46163=DIRECTION('center_axis',(3.66113466765123E-16,1.,-5.66153840231349E-16));
#46164=DIRECTION('ref_axis',(-0.996957691137886,3.20870996777813E-16,-0.0779446090567869));
#46165=DIRECTION('center_axis',(-3.66113466765123E-16,-1.,5.66153840231349E-16));
#46166=DIRECTION('ref_axis',(-0.996957691137886,3.20870996777813E-16,-0.0779446090567869));
#46167=DIRECTION('center_axis',(3.66113466765123E-16,1.,-5.66153840231349E-16));
#46168=DIRECTION('ref_axis',(-0.996957691137886,3.20870996777813E-16,-0.0779446090567869));
#46169=DIRECTION('center_axis',(-3.66113466765123E-16,-1.,5.66153840231349E-16));
#46170=DIRECTION('ref_axis',(-0.996957691137886,3.20870996777813E-16,-0.0779446090567869));
#46171=DIRECTION('center_axis',(3.66113466765123E-16,1.,-5.66153840231349E-16));
#46172=DIRECTION('ref_axis',(-0.996957691137886,3.20870996777813E-16,-0.0779446090567869));
#46173=DIRECTION('center_axis',(-3.66113466765123E-16,-1.,5.66153840231349E-16));
#46174=DIRECTION('ref_axis',(-0.996957691137886,3.20870996777813E-16,-0.0779446090567869));
#46175=DIRECTION('center_axis',(3.66113466765123E-16,1.,-5.66153840231349E-16));
#46176=DIRECTION('ref_axis',(-0.996957691137886,3.20870996777813E-16,-0.0779446090567869));
#46177=DIRECTION('center_axis',(-3.66113466765123E-16,-1.,5.66153840231349E-16));
#46178=DIRECTION('ref_axis',(-0.996957691137886,3.20870996777813E-16,-0.0779446090567869));
#46179=DIRECTION('center_axis',(3.66113466765123E-16,1.,-5.66153840231349E-16));
#46180=DIRECTION('ref_axis',(-0.996957691137886,3.20870996777813E-16,-0.0779446090567869));
#46181=DIRECTION('center_axis',(-3.66113466765123E-16,-1.,5.66153840231349E-16));
#46182=DIRECTION('ref_axis',(-0.996957691137886,3.20870996777813E-16,-0.0779446090567869));
#46183=DIRECTION('center_axis',(3.66113466765123E-16,1.,-5.66153840231349E-16));
#46184=DIRECTION('ref_axis',(-0.996957691137886,3.20870996777813E-16,-0.0779446090567869));
#46185=DIRECTION('center_axis',(-3.66113466765123E-16,-1.,5.66153840231349E-16));
#46186=DIRECTION('ref_axis',(-0.996957691137886,3.20870996777813E-16,-0.0779446090567869));
#46187=DIRECTION('center_axis',(3.66113466765123E-16,1.,-5.66153840231349E-16));
#46188=DIRECTION('ref_axis',(-0.996957691137886,3.20870996777813E-16,-0.0779446090567869));
#46189=DIRECTION('center_axis',(-3.66113466765123E-16,-1.,5.66153840231349E-16));
#46190=DIRECTION('ref_axis',(-0.996957691137886,3.20870996777813E-16,-0.0779446090567869));
#46191=DIRECTION('center_axis',(3.66113466765123E-16,1.,-5.66153840231349E-16));
#46192=DIRECTION('ref_axis',(-0.996957691137886,3.20870996777813E-16,-0.0779446090567869));
#46193=DIRECTION('center_axis',(-3.66113466765123E-16,-1.,5.66153840231349E-16));
#46194=DIRECTION('ref_axis',(-0.996957691137886,3.20870996777813E-16,-0.0779446090567869));
#46195=DIRECTION('center_axis',(3.66113466765123E-16,1.,-5.66153840231349E-16));
#46196=DIRECTION('ref_axis',(-0.996957691137886,3.20870996777813E-16,-0.0779446090567869));
#46197=DIRECTION('center_axis',(-3.66113466765123E-16,-1.,5.66153840231349E-16));
#46198=DIRECTION('ref_axis',(-0.996957691137886,3.20870996777813E-16,-0.0779446090567869));
#46199=DIRECTION('center_axis',(3.66113466765123E-16,1.,-5.66153840231349E-16));
#46200=DIRECTION('ref_axis',(-0.996957691137886,3.20870996777813E-16,-0.0779446090567869));
#46201=DIRECTION('center_axis',(-3.66113466765123E-16,-1.,5.66153840231349E-16));
#46202=DIRECTION('ref_axis',(-0.996957691137886,3.20870996777813E-16,-0.0779446090567869));
#46203=DIRECTION('center_axis',(3.66113466765123E-16,1.,-5.66153840231349E-16));
#46204=DIRECTION('ref_axis',(-0.996957691137886,3.20870996777813E-16,-0.0779446090567869));
#46205=DIRECTION('center_axis',(-3.66113466765123E-16,-1.,5.66153840231349E-16));
#46206=DIRECTION('ref_axis',(-0.996957691137886,3.20870996777813E-16,-0.0779446090567869));
#46207=DIRECTION('center_axis',(3.66113466765123E-16,1.,-5.66153840231349E-16));
#46208=DIRECTION('ref_axis',(-0.996957691137886,3.20870996777813E-16,-0.0779446090567869));
#46209=DIRECTION('center_axis',(-3.66113466765123E-16,-1.,5.66153840231349E-16));
#46210=DIRECTION('ref_axis',(-0.996957691137886,3.20870996777813E-16,-0.0779446090567869));
#46211=DIRECTION('center_axis',(3.66113466765123E-16,1.,-5.66153840231349E-16));
#46212=DIRECTION('ref_axis',(-0.996957691137886,3.20870996777813E-16,-0.0779446090567869));
#46213=DIRECTION('center_axis',(-3.66113466765123E-16,-1.,5.66153840231349E-16));
#46214=DIRECTION('ref_axis',(-0.996957691137886,3.20870996777813E-16,-0.0779446090567869));
#46215=DIRECTION('center_axis',(3.66113466765123E-16,1.,-5.66153840231349E-16));
#46216=DIRECTION('ref_axis',(-0.996957691137886,3.20870996777813E-16,-0.0779446090567869));
#46217=DIRECTION('center_axis',(-3.66113466765123E-16,-1.,5.66153840231349E-16));
#46218=DIRECTION('ref_axis',(-0.996957691137886,3.20870996777813E-16,-0.0779446090567869));
#46219=DIRECTION('center_axis',(3.66113466765123E-16,1.,-5.66153840231349E-16));
#46220=DIRECTION('ref_axis',(-0.996957691137886,3.20870996777813E-16,-0.0779446090567869));
#46221=DIRECTION('center_axis',(-3.66113466765123E-16,-1.,5.66153840231349E-16));
#46222=DIRECTION('ref_axis',(-0.996957691137886,3.20870996777813E-16,-0.0779446090567869));
#46223=DIRECTION('center_axis',(3.66113466765123E-16,1.,-5.66153840231349E-16));
#46224=DIRECTION('ref_axis',(-0.996957691137886,3.20870996777813E-16,-0.0779446090567869));
#46225=DIRECTION('center_axis',(-3.66113466765123E-16,-1.,5.66153840231349E-16));
#46226=DIRECTION('ref_axis',(-0.996957691137886,3.20870996777813E-16,-0.0779446090567869));
#46227=DIRECTION('center_axis',(3.66113466765123E-16,1.,-5.66153840231349E-16));
#46228=DIRECTION('ref_axis',(-0.996957691137886,3.20870996777813E-16,-0.0779446090567869));
#46229=DIRECTION('center_axis',(-3.66113466765123E-16,-1.,5.66153840231349E-16));
#46230=DIRECTION('ref_axis',(-0.996957691137886,3.20870996777813E-16,-0.0779446090567869));
#46231=DIRECTION('center_axis',(3.66113466765123E-16,1.,-5.66153840231349E-16));
#46232=DIRECTION('ref_axis',(-0.996957691137886,3.20870996777813E-16,-0.0779446090567869));
#46233=DIRECTION('center_axis',(-3.66113466765123E-16,-1.,5.66153840231349E-16));
#46234=DIRECTION('ref_axis',(-0.996957691137886,3.20870996777813E-16,-0.0779446090567869));
#46235=DIRECTION('center_axis',(3.66113466765123E-16,1.,-5.66153840231349E-16));
#46236=DIRECTION('ref_axis',(-0.996957691137886,3.20870996777813E-16,-0.0779446090567869));
#46237=DIRECTION('center_axis',(-3.66113466765123E-16,-1.,5.66153840231349E-16));
#46238=DIRECTION('ref_axis',(-0.996957691137886,3.20870996777813E-16,-0.0779446090567869));
#46239=DIRECTION('center_axis',(3.66113466765123E-16,1.,-5.66153840231349E-16));
#46240=DIRECTION('ref_axis',(-0.996957691137886,3.20870996777813E-16,-0.0779446090567869));
#46241=DIRECTION('center_axis',(-3.66113466765123E-16,-1.,5.66153840231349E-16));
#46242=DIRECTION('ref_axis',(-0.996957691137886,3.20870996777813E-16,-0.0779446090567869));
#46243=DIRECTION('center_axis',(3.66113466765123E-16,1.,-5.66153840231349E-16));
#46244=DIRECTION('ref_axis',(-0.996957691137886,3.20870996777813E-16,-0.0779446090567869));
#46245=DIRECTION('center_axis',(-3.66113466765123E-16,-1.,5.66153840231349E-16));
#46246=DIRECTION('ref_axis',(-0.996957691137886,3.20870996777813E-16,-0.0779446090567869));
#46247=DIRECTION('center_axis',(3.66113466765123E-16,1.,-5.66153840231349E-16));
#46248=DIRECTION('ref_axis',(-0.996957691137886,3.20870996777813E-16,-0.0779446090567869));
#46249=DIRECTION('center_axis',(-3.66113466765123E-16,-1.,5.66153840231349E-16));
#46250=DIRECTION('ref_axis',(-0.996957691137886,3.20870996777813E-16,-0.0779446090567869));
#46251=DIRECTION('center_axis',(3.66113466765123E-16,1.,-5.66153840231349E-16));
#46252=DIRECTION('ref_axis',(-0.996957691137886,3.20870996777813E-16,-0.0779446090567869));
#46253=DIRECTION('center_axis',(-3.66113466765123E-16,-1.,5.66153840231349E-16));
#46254=DIRECTION('ref_axis',(-0.996957691137886,3.20870996777813E-16,-0.0779446090567869));
#46255=DIRECTION('center_axis',(3.66113466765123E-16,1.,-5.66153840231349E-16));
#46256=DIRECTION('ref_axis',(-0.996957691137886,3.20870996777813E-16,-0.0779446090567869));
#46257=DIRECTION('center_axis',(-3.66113466765123E-16,-1.,5.66153840231349E-16));
#46258=DIRECTION('ref_axis',(-0.996957691137886,3.20870996777813E-16,-0.0779446090567869));
#46259=DIRECTION('center_axis',(3.66113466765123E-16,1.,-5.66153840231349E-16));
#46260=DIRECTION('ref_axis',(-0.996957691137886,3.20870996777813E-16,-0.0779446090567869));
#46261=DIRECTION('center_axis',(-3.66113466765123E-16,-1.,5.66153840231349E-16));
#46262=DIRECTION('ref_axis',(-0.996957691137886,3.20870996777813E-16,-0.0779446090567869));
#46263=DIRECTION('center_axis',(3.66113466765123E-16,1.,-5.66153840231349E-16));
#46264=DIRECTION('ref_axis',(-0.0201496574551477,-5.58661835927051E-16,
-0.999796975042654));
#46265=DIRECTION('',(3.66113466765123E-16,1.,-5.66153840231349E-16));
#46266=DIRECTION('center_axis',(-3.66113466765123E-16,-1.,5.66153840231349E-16));
#46267=DIRECTION('ref_axis',(-0.0201496574551477,-5.58661835927051E-16,
-0.999796975042654));
#46268=DIRECTION('',(3.66113466765123E-16,1.,-5.66153840231349E-16));
#46269=DIRECTION('center_axis',(3.66113466765123E-16,1.,-5.66153840231349E-16));
#46270=DIRECTION('ref_axis',(0.883011221719068,-5.89007665877645E-16,-0.469351874736002));
#46271=DIRECTION('center_axis',(-3.66113466765123E-16,-1.,5.66153840231349E-16));
#46272=DIRECTION('ref_axis',(0.883011221719068,-5.89007665877645E-16,-0.469351874736002));
#46273=DIRECTION('',(-3.66113466765123E-16,-1.,5.66153840231349E-16));
#46274=DIRECTION('center_axis',(3.66113466765123E-16,1.,-5.66153840231349E-16));
#46275=DIRECTION('ref_axis',(-0.963351194554152,2.00828862743045E-16,-0.268243314830189));
#46276=DIRECTION('center_axis',(-3.66113466765123E-16,-1.,5.66153840231349E-16));
#46277=DIRECTION('ref_axis',(-0.963351194554152,2.00828862743045E-16,-0.268243314830189));
#46278=DIRECTION('center_axis',(3.66113466765123E-16,1.,-5.66153840231349E-16));
#46279=DIRECTION('ref_axis',(-0.996957691137886,3.20870996777813E-16,-0.0779446090567869));
#46280=DIRECTION('center_axis',(-3.66113466765123E-16,-1.,5.66153840231349E-16));
#46281=DIRECTION('ref_axis',(-0.996957691137886,3.20870996777813E-16,-0.0779446090567869));
#46282=DIRECTION('center_axis',(-3.66113466765123E-16,-1.,5.66153840231349E-16));
#46283=DIRECTION('ref_axis',(-0.996957691137886,3.20870996777813E-16,-0.0779446090567869));
#57600=CARTESIAN_POINT('',(0.,0.,0.));
#57601=CARTESIAN_POINT('Origin',(375.115917770968,8.52799273120997,445.000000551893));
#57602=CARTESIAN_POINT('',(347.201102419107,10.52799273121,442.817551498303));
#57603=CARTESIAN_POINT('Origin',(375.115917770968,10.52799273121,445.000000551893));
#57604=CARTESIAN_POINT('',(345.207187036831,8.52799273120998,442.661662280189));
#57605=CARTESIAN_POINT('Origin',(347.201102419107,8.52799273120997,442.817551498303));
#57606=CARTESIAN_POINT('',(405.024648505105,8.52799273120996,447.338338823596));
#57607=CARTESIAN_POINT('Origin',(375.115917770968,8.52799273120997,445.000000551893));
#57608=CARTESIAN_POINT('Origin',(375.115917770968,8.52799273120997,445.000000551893));
#57609=CARTESIAN_POINT('Origin',(375.115917770968,0.527992731209963,445.000000551893));
#57610=CARTESIAN_POINT('',(405.024648505105,2.52799273120996,447.338338823596));
#57611=CARTESIAN_POINT('',(405.024648505105,0.527992731209953,447.338338823596));
#57612=CARTESIAN_POINT('Origin',(375.115917770968,2.52799273120996,445.000000551893));
#57613=CARTESIAN_POINT('Origin',(375.115917770968,10.52799273121,445.000000551893));
#57614=CARTESIAN_POINT('',(370.20573283719,10.52799273121,430.826430644628));
#57615=CARTESIAN_POINT('',(370.61511919622,10.52799273121,425.590136765932));
#57616=CARTESIAN_POINT('',(369.87464541018,10.52799273121,435.061234831742));
#57617=CARTESIAN_POINT('',(382.578611489874,10.52799273121,426.525472074613));
#57618=CARTESIAN_POINT('',(379.587738416461,10.52799273121,426.291638247443));
#57619=CARTESIAN_POINT('',(382.169225130845,10.52799273121,431.76176595331));
#57620=CARTESIAN_POINT('',(381.63344452432,10.52799273121,438.614717079772));
#57621=CARTESIAN_POINT('Origin',(375.115917770968,10.52799273121,445.000000551893));
#57622=CARTESIAN_POINT('Origin',(375.115917770968,2.52799273120996,445.000000551893));
#57623=CARTESIAN_POINT('',(407.018563887381,0.527992731209954,447.49422804171));
#57624=CARTESIAN_POINT('Origin',(375.115917770968,0.527992731209963,445.000000551893));
#57625=CARTESIAN_POINT('Origin',(407.01856388738,2.52799273120995,447.49422804171));
#57626=CARTESIAN_POINT('Origin',(375.115917770968,0.527992731209963,445.000000551893));
#57627=CARTESIAN_POINT('',(369.955795828192,0.527992731209939,392.88413862239));
#57628=CARTESIAN_POINT('',(368.669502598942,0.527992731209941,398.570383318602));
#57629=CARTESIAN_POINT('Origin',(395.540875463479,0.527992731209934,401.660384084767));
#57630=CARTESIAN_POINT('',(366.851654333074,0.527992731209943,398.859263942806));
#57631=CARTESIAN_POINT('Origin',(375.115917770968,0.527992731209963,445.000000551893));
#57632=CARTESIAN_POINT('',(363.86600065809,0.527992731209941,393.851889266405));
#57633=CARTESIAN_POINT('Origin',(342.261939664104,0.527992731209959,410.127126067386));
#57634=CARTESIAN_POINT('',(361.866608510987,0.527992731209941,394.332992279718));
#57635=CARTESIAN_POINT('Origin',(375.115917770968,0.527992731209963,445.000000551893));
#57636=CARTESIAN_POINT('',(361.48567633301,0.527992731209945,400.150450461139));
#57637=CARTESIAN_POINT('Origin',(388.509600623927,0.527992731209934,398.99879935135));
#57638=CARTESIAN_POINT('',(359.735399681749,0.527992731209945,400.720148606485));
#57639=CARTESIAN_POINT('Origin',(375.115917770968,0.527992731209963,445.000000551893));
#57640=CARTESIAN_POINT('',(356.003178379154,0.527992731209945,396.241482157054));
#57641=CARTESIAN_POINT('Origin',(337.211107188252,0.527992731209961,415.695963510098));
#57642=CARTESIAN_POINT('',(354.103663159699,0.527992731209945,397.029435834866));
#57643=CARTESIAN_POINT('Origin',(375.115917770968,0.527992731209963,445.000000551893));
#57644=CARTESIAN_POINT('',(354.637471847458,0.52799273120995,402.834862374034));
#57645=CARTESIAN_POINT('Origin',(381.148528861449,0.527992731209936,397.469916860725));
#57646=CARTESIAN_POINT('',(352.997864430793,0.52799273120995,403.671350181463));
#57647=CARTESIAN_POINT('Origin',(375.115917770968,0.527992731209963,445.000000551893));
#57648=CARTESIAN_POINT('',(348.610975175589,0.52799273120995,399.831671590828));
#57649=CARTESIAN_POINT('Origin',(333.0936169478,0.527992731209967,421.986363599303));
#57650=CARTESIAN_POINT('',(346.858109252615,0.52799273120995,400.907073898524));
#57651=CARTESIAN_POINT('Origin',(375.115917770968,0.527992731209963,445.000000551893));
#57652=CARTESIAN_POINT('',(348.293514664609,0.527992731209954,406.557519926939));
#57653=CARTESIAN_POINT('Origin',(373.638914192836,0.527992731209939,397.11138277388));
#57654=CARTESIAN_POINT('',(346.804949058683,0.527992731209954,407.640200290488));
#57655=CARTESIAN_POINT('Origin',(375.115917770968,0.527992731209963,445.000000551893));
#57656=CARTESIAN_POINT('',(341.871411623583,0.527992731209954,404.534055188714));
#57657=CARTESIAN_POINT('Origin',(330.010855217635,0.527992731209972,428.843435808162));
#57658=CARTESIAN_POINT('',(340.308356373543,0.527992731209956,405.870426152421));
#57659=CARTESIAN_POINT('Origin',(375.115917770968,0.527992731209963,445.000000551893));
#57660=CARTESIAN_POINT('',(342.61001406469,0.527992731209959,411.226758936108));
#57661=CARTESIAN_POINT('Origin',(366.16566825421,0.527992731209941,397.93202538994));
#57662=CARTESIAN_POINT('',(341.309143694988,0.527992731209959,412.528972672017));
#57663=CARTESIAN_POINT('Origin',(375.115917770968,0.527992731209963,445.000000551893));
#57664=CARTESIAN_POINT('',(335.950438145117,0.527992731209961,410.232844660214));
#57665=CARTESIAN_POINT('Origin',(328.038729822654,0.527992731209976,436.098336261576));
#57666=CARTESIAN_POINT('',(334.615681175749,0.527992731209961,411.797278391646));
#57667=CARTESIAN_POINT('Origin',(375.115917770968,0.527992731209963,445.000000551893));
#57668=CARTESIAN_POINT('',(337.726916694929,0.527992731209961,416.72760724082));
#57669=CARTESIAN_POINT('Origin',(358.912807162862,0.527992731209945,399.911637764141));
#57670=CARTESIAN_POINT('',(336.645773307294,0.527992731209963,418.217289525112));
#57671=CARTESIAN_POINT('Origin',(375.115917770968,0.527992731209963,445.000000551893));
#57672=CARTESIAN_POINT('',(330.993848757813,0.527992731209963,416.787716895342));
#57673=CARTESIAN_POINT('Origin',(327.225801035189,0.527992731209981,443.572425232748));
#57674=CARTESIAN_POINT('',(329.920256215508,0.527992731209963,418.541691843973));
#57675=CARTESIAN_POINT('Origin',(375.115917770968,0.527992731209963,445.000000551893));
#57676=CARTESIAN_POINT('',(333.764460618641,0.527992731209967,422.924615699545));
#57677=CARTESIAN_POINT('Origin',(352.058920429727,0.52799273120995,403.001475269873));
#57678=CARTESIAN_POINT('',(332.929665551385,0.527992731209967,424.565085610408));
#57679=CARTESIAN_POINT('Origin',(375.115917770968,0.527992731209963,445.000000551893));
#57680=CARTESIAN_POINT('',(327.123691142365,0.527992731209967,424.037269185296));
#57681=CARTESIAN_POINT('Origin',(327.592085859944,0.527992731209985,451.081665846128));
#57682=CARTESIAN_POINT('',(326.337698438563,0.527992731209972,425.937596666782));
#57683=CARTESIAN_POINT('Origin',(375.115917770968,0.527992731209963,445.000000551893));
#57684=CARTESIAN_POINT('',(330.820214655061,0.527992731209972,429.665193397337));
#57685=CARTESIAN_POINT('Origin',(345.77277349292,0.527992731209954,407.125455853163));
#57686=CARTESIAN_POINT('',(330.252323333266,0.527992731209972,431.416057121158));
#57687=CARTESIAN_POINT('Origin',(375.115917770968,0.527992731209963,445.000000551893));
#57688=CARTESIAN_POINT('',(324.435261423582,0.527992731209972,431.802993492812));
#57689=CARTESIAN_POINT('Origin',(329.128565148903,0.52799273120999,458.441155676074));
#57690=CARTESIAN_POINT('',(323.956222307212,0.527992731209976,433.802881137733));
#57691=CARTESIAN_POINT('Origin',(375.115917770968,0.527992731209963,445.000000551893));
#57692=CARTESIAN_POINT('',(328.966675911205,0.527992731209976,436.783364940581));
#57693=CARTESIAN_POINT('Origin',(340.209152152551,0.527992731209959,412.182033425343));
#57694=CARTESIAN_POINT('',(328.679671703937,0.527992731209976,438.601510401696));
#57695=CARTESIAN_POINT('Origin',(375.115917770968,0.527992731209963,445.000000551893));
#57696=CARTESIAN_POINT('',(322.994757663527,0.527992731209981,439.893671912479));
#57697=CARTESIAN_POINT('Origin',(331.797405682692,0.52799273120999,465.469679658226));
#57698=CARTESIAN_POINT('',(322.834467667472,0.527992731209981,441.943875849769));
#57699=CARTESIAN_POINT('Origin',(375.115917770968,0.527992731209963,445.000000551893));
#57700=CARTESIAN_POINT('',(328.249484662489,0.527992731209981,444.103857322026));
#57701=CARTESIAN_POINT('Origin',(335.50505123062,0.527992731209963,418.046698264767));
#57702=CARTESIAN_POINT('',(328.250434565844,0.527992731209981,445.944515745103));
#57703=CARTESIAN_POINT('Origin',(375.115917770968,0.527992731209963,445.000000551893));
#57704=CARTESIAN_POINT('',(322.837649845529,0.527992731209985,448.11008509018));
#57705=CARTESIAN_POINT('Origin',(335.532891749993,0.527992731209994,471.994172205811));
#57706=CARTESIAN_POINT('',(323.000055841466,0.527992731209985,450.160122494669));
#57707=CARTESIAN_POINT('Origin',(375.115917770968,0.527992731209963,445.000000551893));
#57708=CARTESIAN_POINT('',(328.686300537678,0.527992731209985,451.446415723918));
#57709=CARTESIAN_POINT('Origin',(331.776301303842,0.527992731209967,424.575042859381));
#57710=CARTESIAN_POINT('',(328.975181161882,0.527992731209985,453.264263989787));
#57711=CARTESIAN_POINT('Origin',(375.115917770968,0.527992731209963,445.000000551893));
#57712=CARTESIAN_POINT('',(323.96780648548,0.52799273120999,456.24991766477));
#57713=CARTESIAN_POINT('Origin',(340.243043286462,0.527992731209994,477.853978658756));
#57714=CARTESIAN_POINT('',(324.448909498793,0.52799273120999,458.249309811874));
#57715=CARTESIAN_POINT('Origin',(375.115917770968,0.527992731209963,445.000000551893));
#57716=CARTESIAN_POINT('',(330.266367680215,0.527992731209985,458.630241989851));
#57717=CARTESIAN_POINT('Origin',(329.114716570426,0.527992731209972,431.606317698934));
#57718=CARTESIAN_POINT('',(330.836065825561,0.52799273120999,460.380518641112));
#57719=CARTESIAN_POINT('Origin',(375.115917770968,0.527992731209963,445.000000551893));
#57720=CARTESIAN_POINT('',(326.357399376129,0.52799273120999,464.112739943707));
#57721=CARTESIAN_POINT('Origin',(345.811880729174,0.527992731209994,482.904811134609));
#57722=CARTESIAN_POINT('',(327.145353053941,0.527992731209994,466.012255163162));
#57723=CARTESIAN_POINT('Origin',(375.115917770968,0.527992731209963,445.000000551893));
#57724=CARTESIAN_POINT('',(332.95077959311,0.52799273120999,465.478446475402));
#57725=CARTESIAN_POINT('Origin',(327.5858340798,0.527992731209976,438.967389461411));
#57726=CARTESIAN_POINT('',(333.787267400539,0.52799273120999,467.118053892068));
#57727=CARTESIAN_POINT('Origin',(375.115917770968,0.527992731209963,445.000000551893));
#57728=CARTESIAN_POINT('',(329.947588809904,0.527992731209994,471.504943147272));
#57729=CARTESIAN_POINT('Origin',(352.102280818378,0.527992731209994,487.022301375061));
#57730=CARTESIAN_POINT('',(331.022991117599,0.527992731209994,473.257809070246));
#57731=CARTESIAN_POINT('Origin',(375.115917770968,0.527992731209963,445.000000551893));
#57732=CARTESIAN_POINT('',(336.673437146014,0.527992731209994,471.822403658252));
#57733=CARTESIAN_POINT('Origin',(327.227299992955,0.527992731209981,446.477004130025));
#57734=CARTESIAN_POINT('',(337.756117509564,0.527992731209994,473.310969264178));
#57735=CARTESIAN_POINT('Origin',(375.115917770968,0.527992731209963,445.000000551893));
#57736=CARTESIAN_POINT('',(334.64997240779,0.527992731209999,478.244506699278));
#57737=CARTESIAN_POINT('Origin',(358.959353027238,0.527992731209994,490.105063105225));
#57738=CARTESIAN_POINT('',(335.986343371497,0.527992731209999,479.807561949318));
#57739=CARTESIAN_POINT('Origin',(375.115917770968,0.527992731209963,445.000000551893));
#57740=CARTESIAN_POINT('',(341.342676155183,0.527992731209994,477.505904258171));
#57741=CARTESIAN_POINT('Origin',(328.047942609015,0.527992731209985,453.95025006865));
#57742=CARTESIAN_POINT('',(342.644889891093,0.527992731209994,478.806774627873));
#57743=CARTESIAN_POINT('Origin',(375.115917770968,0.527992731209963,445.000000551893));
#57744=CARTESIAN_POINT('',(340.34876187929,0.527992731209999,484.165480177744));
#57745=CARTESIAN_POINT('Origin',(366.214253480652,0.527992731209994,492.077188500207));
#57746=CARTESIAN_POINT('',(341.913195610722,0.527992731209999,485.500237147112));
#57747=CARTESIAN_POINT('Origin',(375.115917770968,0.527992731209963,445.000000551893));
#57748=CARTESIAN_POINT('',(346.843524459896,0.527992731209994,482.389001627931));
#57749=CARTESIAN_POINT('Origin',(330.027554983216,0.52799273120999,461.203111159998));
#57750=CARTESIAN_POINT('',(348.333206744188,0.527992731209994,483.470145015567));
#57751=CARTESIAN_POINT('Origin',(375.115917770968,0.527992731209963,445.000000551893));
#57752=CARTESIAN_POINT('',(346.903634114418,0.527992731209999,489.122069565048));
#57753=CARTESIAN_POINT('Origin',(373.688342451824,0.52799273120999,492.890117287672));
#57754=CARTESIAN_POINT('',(348.657609063049,0.527992731209999,490.195662107353));
#57755=CARTESIAN_POINT('Origin',(375.115917770968,0.527992731209963,445.000000551893));
#57756=CARTESIAN_POINT('',(353.040532918621,0.527992731209994,486.35145770422));
#57757=CARTESIAN_POINT('Origin',(333.117392488949,0.52799273120999,468.056997893134));
#57758=CARTESIAN_POINT('',(354.681002829484,0.527992731209994,487.186252771476));
#57759=CARTESIAN_POINT('Origin',(375.115917770968,0.527992731209963,445.000000551893));
#57760=CARTESIAN_POINT('',(354.153186404372,0.527992731209999,492.992227180495));
#57761=CARTESIAN_POINT('Origin',(381.197583065204,0.52799273120999,492.523832462917));
#57762=CARTESIAN_POINT('',(356.053513885857,0.527992731209999,493.778219884297));
#57763=CARTESIAN_POINT('Origin',(375.115917770968,0.527992731209963,445.000000551893));
#57764=CARTESIAN_POINT('',(359.781110616413,0.527992731209994,489.2957036678));
#57765=CARTESIAN_POINT('Origin',(337.241373072239,0.527992731209994,474.343144829941));
#57766=CARTESIAN_POINT('',(361.531974340233,0.527992731209994,489.863594989594));
#57767=CARTESIAN_POINT('Origin',(375.115917770968,0.527992731209963,445.000000551893));
#57768=CARTESIAN_POINT('',(361.918910711888,0.527992731209999,495.680656899279));
#57769=CARTESIAN_POINT('Origin',(388.55707289515,0.527992731209985,490.987353173957));
#57770=CARTESIAN_POINT('',(363.918798356808,0.527992731209994,496.159696015649));
#57771=CARTESIAN_POINT('Origin',(375.115917770968,0.527992731209963,445.000000551893));
#57772=CARTESIAN_POINT('',(366.899282159657,0.527992731209994,491.149242411656));
#57773=CARTESIAN_POINT('Origin',(342.297950644419,0.527992731209994,479.90676617031));
#57774=CARTESIAN_POINT('',(368.717427620771,0.52799273120999,491.436246618923));
#57775=CARTESIAN_POINT('Origin',(375.115917770968,0.527992731209963,445.000000551893));
#57776=CARTESIAN_POINT('',(370.009589131554,0.527992731209994,497.121160659334));
#57777=CARTESIAN_POINT('Origin',(395.585596877302,0.527992731209981,488.318512640169));
#57778=CARTESIAN_POINT('',(372.059793068845,0.527992731209994,497.281450655388));
#57779=CARTESIAN_POINT('Origin',(375.115917770968,0.527992731209963,445.000000551893));
#57780=CARTESIAN_POINT('',(374.219774541101,0.52799273120999,491.866433660372));
#57781=CARTESIAN_POINT('Origin',(348.162615483842,0.527992731209994,484.61086709224));
#57782=CARTESIAN_POINT('',(376.060432964178,0.52799273120999,491.865483757017));
#57783=CARTESIAN_POINT('Origin',(375.115917770968,0.527992731209963,445.000000551893));
#57784=CARTESIAN_POINT('',(378.226002309256,0.52799273120999,497.278268477331));
#57785=CARTESIAN_POINT('Origin',(402.110089424886,0.527992731209976,484.583026572868));
#57786=CARTESIAN_POINT('',(380.276039713744,0.52799273120999,497.115862481395));
#57787=CARTESIAN_POINT('Origin',(375.115917770968,0.527992731209963,445.000000551893));
#57788=CARTESIAN_POINT('',(381.562332942994,0.527992731209985,491.429617785183));
#57789=CARTESIAN_POINT('Origin',(354.690960078457,0.527992731209994,488.339617019018));
#57790=CARTESIAN_POINT('',(383.380181208862,0.527992731209985,491.140737160979));
#57791=CARTESIAN_POINT('Origin',(375.115917770968,0.527992731209963,445.000000551893));
#57792=CARTESIAN_POINT('',(386.365834883846,0.52799273120999,496.14811183738));
#57793=CARTESIAN_POINT('Origin',(407.969895877832,0.527992731209972,479.872875036399));
#57794=CARTESIAN_POINT('',(388.365227030949,0.527992731209985,495.667008824067));
#57795=CARTESIAN_POINT('Origin',(375.115917770968,0.527992731209963,445.000000551893));
#57796=CARTESIAN_POINT('',(388.746159208926,0.527992731209985,489.849550642646));
#57797=CARTESIAN_POINT('Origin',(361.72223491801,0.527992731209994,491.001201752435));
#57798=CARTESIAN_POINT('',(390.496435860187,0.527992731209981,489.2798524973));
#57799=CARTESIAN_POINT('Origin',(375.115917770968,0.527992731209963,445.000000551893));
#57800=CARTESIAN_POINT('',(394.228657162783,0.527992731209985,493.758518946731));
#57801=CARTESIAN_POINT('Origin',(413.020728353684,0.527992731209967,474.304037593687));
#57802=CARTESIAN_POINT('',(396.128172382238,0.527992731209981,492.970565268919));
#57803=CARTESIAN_POINT('Origin',(375.115917770968,0.527992731209963,445.000000551893));
#57804=CARTESIAN_POINT('',(395.594363694478,0.527992731209981,487.165138729751));
#57805=CARTESIAN_POINT('Origin',(369.083306680487,0.527992731209994,492.53008424306));
#57806=CARTESIAN_POINT('',(397.233971111143,0.527992731209976,486.328650922322));
#57807=CARTESIAN_POINT('Origin',(375.115917770968,0.527992731209963,445.000000551893));
#57808=CARTESIAN_POINT('',(401.620860366348,0.527992731209981,490.168329512957));
#57809=CARTESIAN_POINT('Origin',(417.138218594136,0.527992731209961,468.013637504482));
#57810=CARTESIAN_POINT('',(403.373726289321,0.527992731209976,489.092927205261));
#57811=CARTESIAN_POINT('Origin',(375.115917770968,0.527992731209963,445.000000551893));
#57812=CARTESIAN_POINT('',(401.938320877327,0.527992731209976,483.442481176847));
#57813=CARTESIAN_POINT('Origin',(376.5929213491,0.52799273120999,492.888618329905));
#57814=CARTESIAN_POINT('',(403.426886483253,0.527992731209972,482.359800813297));
#57815=CARTESIAN_POINT('Origin',(375.115917770968,0.527992731209963,445.000000551893));
#57816=CARTESIAN_POINT('',(408.360423918353,0.527992731209972,485.465945915071));
#57817=CARTESIAN_POINT('Origin',(420.220980324301,0.527992731209959,461.156565295623));
#57818=CARTESIAN_POINT('',(409.923479168393,0.527992731209972,484.129574951364));
#57819=CARTESIAN_POINT('Origin',(375.115917770968,0.527992731209963,445.000000551893));
#57820=CARTESIAN_POINT('',(407.621821477246,0.527992731209972,478.773242167677));
#57821=CARTESIAN_POINT('Origin',(384.066167287726,0.527992731209985,492.067975713845));
#57822=CARTESIAN_POINT('',(408.922691846948,0.527992731209967,477.471028431768));
#57823=CARTESIAN_POINT('Origin',(375.115917770968,0.527992731209963,445.000000551893));
#57824=CARTESIAN_POINT('',(414.28139739682,0.527992731209967,479.767156443571));
#57825=CARTESIAN_POINT('Origin',(422.193105719283,0.527992731209954,453.901664842209));
#57826=CARTESIAN_POINT('',(415.616154366188,0.527992731209967,478.202722712139));
#57827=CARTESIAN_POINT('Origin',(375.115917770968,0.527992731209963,445.000000551893));
#57828=CARTESIAN_POINT('',(412.504918847007,0.527992731209967,473.272393862965));
#57829=CARTESIAN_POINT('Origin',(391.319028379074,0.527992731209981,490.088363339644));
#57830=CARTESIAN_POINT('',(413.586062234642,0.527992731209963,471.782711578673));
#57831=CARTESIAN_POINT('Origin',(375.115917770968,0.527992731209963,445.000000551893));
#57832=CARTESIAN_POINT('',(419.237986784123,0.527992731209963,473.212284208443));
#57833=CARTESIAN_POINT('Origin',(423.006034506748,0.527992731209947,446.427575871037));
#57834=CARTESIAN_POINT('',(420.311579326428,0.527992731209963,471.458309259812));
#57835=CARTESIAN_POINT('Origin',(375.115917770968,0.527992731209963,445.000000551893));
#57836=CARTESIAN_POINT('',(416.467374923295,0.527992731209961,467.07538540424));
#57837=CARTESIAN_POINT('Origin',(398.17291511221,0.527992731209976,486.998525833912));
#57838=CARTESIAN_POINT('',(417.302169990551,0.527992731209961,465.434915493377));
#57839=CARTESIAN_POINT('Origin',(375.115917770968,0.527992731209963,445.000000551893));
#57840=CARTESIAN_POINT('',(423.108144399571,0.527992731209959,465.962731918489));
#57841=CARTESIAN_POINT('Origin',(422.639749681993,0.527992731209945,438.918335257657));
#57842=CARTESIAN_POINT('',(423.894137103373,0.527992731209959,464.062404437003));
#57843=CARTESIAN_POINT('Origin',(375.115917770968,0.527992731209963,445.000000551893));
#57844=CARTESIAN_POINT('',(419.411620886875,0.527992731209959,460.334807706448));
#57845=CARTESIAN_POINT('Origin',(404.459062049017,0.527992731209972,482.874545250622));
#57846=CARTESIAN_POINT('',(419.97951220867,0.527992731209956,458.583943982627));
#57847=CARTESIAN_POINT('Origin',(375.115917770968,0.527992731209963,445.000000551893));
#57848=CARTESIAN_POINT('',(425.796574118354,0.527992731209954,458.197007610973));
#57849=CARTESIAN_POINT('Origin',(421.103270393033,0.527992731209941,431.558845427711));
#57850=CARTESIAN_POINT('',(426.275613234725,0.527992731209952,456.197119966052));
#57851=CARTESIAN_POINT('Origin',(375.115917770968,0.527992731209963,445.000000551893));
#57852=CARTESIAN_POINT('',(421.265159630731,0.527992731209952,453.216636163204));
#57853=CARTESIAN_POINT('Origin',(410.022683389386,0.527992731209967,477.817967678442));
#57854=CARTESIAN_POINT('',(421.552163837999,0.527992731209952,451.39849070209));
#57855=CARTESIAN_POINT('Origin',(375.115917770968,0.527992731209963,445.000000551893));
#57856=CARTESIAN_POINT('',(427.23707787841,0.52799273120995,450.106329191307));
#57857=CARTESIAN_POINT('Origin',(418.434429859244,0.527992731209939,424.530321445559));
#57858=CARTESIAN_POINT('',(427.397367874464,0.527992731209947,448.056125254016));
#57859=CARTESIAN_POINT('Origin',(375.115917770968,0.527992731209963,445.000000551893));
#57860=CARTESIAN_POINT('',(421.982350879447,0.52799273120995,445.896143781759));
#57861=CARTESIAN_POINT('Origin',(414.726784311316,0.527992731209963,471.953302839018));
#57862=CARTESIAN_POINT('',(421.981400976092,0.527992731209947,444.055485358683));
#57863=CARTESIAN_POINT('Origin',(375.115917770968,0.527992731209963,445.000000551893));
#57864=CARTESIAN_POINT('',(427.394185696407,0.527992731209945,441.889916013605));
#57865=CARTESIAN_POINT('Origin',(414.698943791944,0.527992731209936,418.005828897974));
#57866=CARTESIAN_POINT('',(427.23177970047,0.527992731209943,439.839878609116));
#57867=CARTESIAN_POINT('Origin',(375.115917770968,0.527992731209963,445.000000551893));
#57868=CARTESIAN_POINT('',(421.545535004259,0.527992731209945,438.553585379867));
#57869=CARTESIAN_POINT('Origin',(418.455534238094,0.527992731209961,465.424958244404));
#57870=CARTESIAN_POINT('',(421.256654380055,0.527992731209943,436.735737113998));
#57871=CARTESIAN_POINT('Origin',(375.115917770968,0.527992731209963,445.000000551893));
#57872=CARTESIAN_POINT('',(426.264029056456,0.527992731209941,433.750083439015));
#57873=CARTESIAN_POINT('Origin',(409.988792255475,0.527992731209934,412.146022445029));
#57874=CARTESIAN_POINT('',(425.782926043143,0.527992731209939,431.750691291911));
#57875=CARTESIAN_POINT('Origin',(375.115917770968,0.527992731209963,445.000000551893));
#57876=CARTESIAN_POINT('',(419.965467861721,0.527992731209941,431.369759113934));
#57877=CARTESIAN_POINT('Origin',(421.117118971511,0.527992731209956,458.393683404851));
#57878=CARTESIAN_POINT('',(419.395769716376,0.527992731209941,429.619482462673));
#57879=CARTESIAN_POINT('Origin',(375.115917770968,0.527992731209963,445.000000551893));
#57880=CARTESIAN_POINT('',(423.874436165807,0.527992731209936,425.887261160078));
#57881=CARTESIAN_POINT('Origin',(404.419954812762,0.527992731209934,407.095189969177));
#57882=CARTESIAN_POINT('',(423.086482487995,0.527992731209936,423.987745940623));
#57883=CARTESIAN_POINT('Origin',(375.115917770968,0.527992731209963,445.000000551893));
#57884=CARTESIAN_POINT('',(417.281055948826,0.527992731209939,424.521554628383));
#57885=CARTESIAN_POINT('Origin',(422.646001462136,0.527992731209952,451.032611642374));
#57886=CARTESIAN_POINT('',(416.444568141397,0.527992731209939,422.881947211718));
#57887=CARTESIAN_POINT('Origin',(375.115917770968,0.527992731209963,445.000000551893));
#57888=CARTESIAN_POINT('',(420.284246732032,0.527992731209934,418.495057956513));
#57889=CARTESIAN_POINT('Origin',(398.129554723558,0.527992731209932,402.977699728725));
#57890=CARTESIAN_POINT('',(419.208844424337,0.527992731209934,416.742192033539));
#57891=CARTESIAN_POINT('Origin',(375.115917770968,0.527992731209963,445.000000551893));
#57892=CARTESIAN_POINT('',(413.558398395922,0.527992731209936,418.177597445533));
#57893=CARTESIAN_POINT('Origin',(423.004535548981,0.527992731209947,443.522996973761));
#57894=CARTESIAN_POINT('',(412.475718032372,0.527992731209936,416.689031839608));
#57895=CARTESIAN_POINT('Origin',(375.115917770968,0.527992731209963,445.000000551893));
#57896=CARTESIAN_POINT('',(415.581863134147,0.527992731209932,411.755494404508));
#57897=CARTESIAN_POINT('Origin',(391.272482514698,0.527992731209934,399.89493799856));
#57898=CARTESIAN_POINT('',(414.245492170439,0.527992731209932,410.192439154467));
#57899=CARTESIAN_POINT('Origin',(375.115917770968,0.527992731209963,445.000000551893));
#57900=CARTESIAN_POINT('',(408.889159386753,0.527992731209934,412.494096845614));
#57901=CARTESIAN_POINT('Origin',(422.183892932921,0.527992731209943,436.049751035135));
#57902=CARTESIAN_POINT('',(407.586945650843,0.527992731209934,411.193226475912));
#57903=CARTESIAN_POINT('Origin',(375.115917770968,0.527992731209963,445.000000551893));
#57904=CARTESIAN_POINT('',(409.883073662646,0.52799273120993,405.834520926041));
#57905=CARTESIAN_POINT('Origin',(384.017582061284,0.527992731209936,397.922812603578));
#57906=CARTESIAN_POINT('',(408.318639931215,0.52799273120993,404.499763956673));
#57907=CARTESIAN_POINT('Origin',(375.115917770968,0.527992731209963,445.000000551893));
#57908=CARTESIAN_POINT('',(403.38831108204,0.527992731209934,407.610999475854));
#57909=CARTESIAN_POINT('Origin',(420.20428055872,0.527992731209939,428.796889943787));
#57910=CARTESIAN_POINT('',(401.898628797749,0.527992731209934,406.529856088218));
#57911=CARTESIAN_POINT('Origin',(375.115917770968,0.527992731209963,445.000000551893));
#57912=CARTESIAN_POINT('',(403.328201427518,0.52799273120993,400.877931538737));
#57913=CARTESIAN_POINT('Origin',(376.543493090113,0.527992731209939,397.109883816113));
#57914=CARTESIAN_POINT('',(401.574226478887,0.52799273120993,399.804338996432));
#57915=CARTESIAN_POINT('Origin',(375.115917770968,0.527992731209963,445.000000551893));
#57916=CARTESIAN_POINT('',(397.191302623315,0.527992731209934,403.648543399565));
#57917=CARTESIAN_POINT('Origin',(417.114443052987,0.527992731209936,421.943003210651));
#57918=CARTESIAN_POINT('',(395.550832712453,0.527992731209934,402.813748332309));
#57919=CARTESIAN_POINT('Origin',(375.115917770968,0.527992731209963,445.000000551893));
#57920=CARTESIAN_POINT('',(396.078649137564,0.52799273120993,397.00777392329));
#57921=CARTESIAN_POINT('Origin',(369.034252476732,0.527992731209941,397.476168640868));
#57922=CARTESIAN_POINT('',(394.178321656079,0.52799273120993,396.221781219488));
#57923=CARTESIAN_POINT('Origin',(375.115917770968,0.527992731209963,445.000000551893));
#57924=CARTESIAN_POINT('',(390.450724925524,0.527992731209934,400.704297435985));
#57925=CARTESIAN_POINT('Origin',(412.990462469698,0.527992731209934,415.656856273844));
#57926=CARTESIAN_POINT('',(388.699861201703,0.527992731209934,400.136406114191));
#57927=CARTESIAN_POINT('Origin',(375.115917770968,0.527992731209963,445.000000551893));
#57928=CARTESIAN_POINT('',(388.312924830048,0.527992731209932,394.319344204506));
#57929=CARTESIAN_POINT('Origin',(361.674762646786,0.527992731209943,399.012647929828));
#57930=CARTESIAN_POINT('',(386.313037185128,0.527992731209932,393.840305088136));
#57931=CARTESIAN_POINT('Origin',(375.115917770968,0.527992731209963,445.000000551893));
#57932=CARTESIAN_POINT('',(383.33255338228,0.527992731209936,398.850758692129));
#57933=CARTESIAN_POINT('Origin',(407.933884897518,0.527992731209934,410.093234933475));
#57934=CARTESIAN_POINT('',(381.514407921165,0.527992731209936,398.563754484862));
#57935=CARTESIAN_POINT('Origin',(375.115917770968,0.527992731209963,445.000000551893));
#57936=CARTESIAN_POINT('',(380.222246410382,0.527992731209934,392.878840444451));
#57937=CARTESIAN_POINT('Origin',(354.646238664634,0.527992731209947,401.681488463616));
#57938=CARTESIAN_POINT('',(378.172042473091,0.527992731209934,392.718550448397));
#57939=CARTESIAN_POINT('Origin',(375.115917770968,0.527992731209963,445.000000551893));
#57940=CARTESIAN_POINT('',(376.012061000835,0.527992731209939,398.133567443413));
#57941=CARTESIAN_POINT('Origin',(402.069220058094,0.527992731209932,405.389134011545));
#57942=CARTESIAN_POINT('',(374.171402577758,0.527992731209939,398.134517346768));
#57943=CARTESIAN_POINT('Origin',(375.115917770968,0.527992731209963,445.000000551893));
#57944=CARTESIAN_POINT('',(372.005833232681,0.527992731209936,392.721732626454));
#57945=CARTESIAN_POINT('Origin',(348.12174611705,0.527992731209952,405.416974530917));
#57946=CARTESIAN_POINT('Origin',(375.115917770968,0.527992731209963,445.000000551893));
#57947=CARTESIAN_POINT('Origin',(370.61511919622,0.527992731209956,425.590136765932));
#57948=CARTESIAN_POINT('',(382.578611489874,-19.4720072687901,426.525472074613));
#57949=CARTESIAN_POINT('',(370.61511919622,-19.47200726879,425.590136765932));
#57950=CARTESIAN_POINT('',(373.605992269633,-19.47200726879,425.823970593102));
#57951=CARTESIAN_POINT('',(382.578611489874,0.527992731209952,426.525472074613));
#57952=CARTESIAN_POINT('',(370.61511919622,0.527992731209956,425.590136765932));
#57953=CARTESIAN_POINT('Origin',(369.991562323765,0.527992731209961,433.565798295035));
#57954=CARTESIAN_POINT('',(370.20573283719,-19.47200726879,430.826430644628));
#57955=CARTESIAN_POINT('',(369.562866973953,-19.47200726879,439.049065596293));
#57956=CARTESIAN_POINT('',(370.20573283719,0.527992731209959,430.826430644628));
#57957=CARTESIAN_POINT('Origin',(375.115917770968,0.527992731209963,445.000000551893));
#57958=CARTESIAN_POINT('',(382.169225130845,-19.47200726879,431.76176595331));
#57959=CARTESIAN_POINT('Origin',(375.115917770968,-19.47200726879,445.000000551893));
#57960=CARTESIAN_POINT('',(382.169225130845,0.527992731209954,431.76176595331));
#57961=CARTESIAN_POINT('Origin',(382.578611489874,0.527992731209952,426.525472074613));
#57962=CARTESIAN_POINT('',(381.838137703835,-19.47200726879,435.996570140423));
#57963=CARTESIAN_POINT('Origin',(375.115917770968,-19.47200726879,445.000000551893));
#57964=CARTESIAN_POINT('',(368.669502598942,-19.4720072687901,398.570383318602));
#57965=CARTESIAN_POINT('',(368.669502598942,-19.4720072687901,398.570383318602));
#57966=CARTESIAN_POINT('',(366.851654333074,-19.4720072687901,398.859263942806));
#57967=CARTESIAN_POINT('Origin',(375.115917770968,-19.47200726879,445.000000551893));
#57968=CARTESIAN_POINT('',(366.851654333074,-19.4720072687901,398.859263942806));
#57969=CARTESIAN_POINT('Origin',(342.261939664104,-19.47200726879,410.127126067386));
#57970=CARTESIAN_POINT('',(363.86600065809,-19.4720072687901,393.851889266405));
#57971=CARTESIAN_POINT('Origin',(342.261939664104,-19.47200726879,410.127126067386));
#57972=CARTESIAN_POINT('',(363.86600065809,-19.4720072687901,393.851889266405));
#57973=CARTESIAN_POINT('Origin',(395.540875463479,-19.4720072687901,401.660384084767));
#57974=CARTESIAN_POINT('',(369.955795828192,-19.4720072687901,392.88413862239));
#57975=CARTESIAN_POINT('',(369.955795828192,-19.4720072687901,392.88413862239));
#57976=CARTESIAN_POINT('Origin',(395.540875463479,-19.4720072687901,401.660384084767));
#57977=CARTESIAN_POINT('Origin',(375.115917770968,-19.47200726879,445.000000551893));
#57978=CARTESIAN_POINT('',(361.48567633301,-19.4720072687901,400.150450461139));
#57979=CARTESIAN_POINT('',(361.48567633301,-19.4720072687901,400.150450461139));
#57980=CARTESIAN_POINT('',(359.735399681749,-19.4720072687901,400.720148606485));
#57981=CARTESIAN_POINT('Origin',(375.115917770968,-19.47200726879,445.000000551893));
#57982=CARTESIAN_POINT('',(359.735399681749,-19.4720072687901,400.720148606485));
#57983=CARTESIAN_POINT('Origin',(337.211107188252,-19.47200726879,415.695963510098));
#57984=CARTESIAN_POINT('',(356.003178379154,-19.4720072687901,396.241482157054));
#57985=CARTESIAN_POINT('Origin',(337.211107188252,-19.47200726879,415.695963510098));
#57986=CARTESIAN_POINT('',(356.003178379154,-19.4720072687901,396.241482157054));
#57987=CARTESIAN_POINT('Origin',(388.509600623927,-19.4720072687901,398.99879935135));
#57988=CARTESIAN_POINT('',(361.866608510987,-19.4720072687901,394.332992279718));
#57989=CARTESIAN_POINT('',(361.866608510987,-19.4720072687901,394.332992279718));
#57990=CARTESIAN_POINT('Origin',(388.509600623927,-19.4720072687901,398.99879935135));
#57991=CARTESIAN_POINT('Origin',(375.115917770968,-19.47200726879,445.000000551893));
#57992=CARTESIAN_POINT('',(354.637471847458,-19.4720072687901,402.834862374034));
#57993=CARTESIAN_POINT('',(354.637471847458,-19.4720072687901,402.834862374034));
#57994=CARTESIAN_POINT('',(352.997864430793,-19.4720072687901,403.671350181463));
#57995=CARTESIAN_POINT('Origin',(375.115917770968,-19.47200726879,445.000000551893));
#57996=CARTESIAN_POINT('',(352.997864430793,-19.4720072687901,403.671350181463));
#57997=CARTESIAN_POINT('Origin',(333.0936169478,-19.47200726879,421.986363599303));
#57998=CARTESIAN_POINT('',(348.610975175589,-19.4720072687901,399.831671590828));
#57999=CARTESIAN_POINT('Origin',(333.0936169478,-19.47200726879,421.986363599303));
#58000=CARTESIAN_POINT('',(348.610975175589,-19.4720072687901,399.831671590828));
#58001=CARTESIAN_POINT('Origin',(381.148528861449,-19.4720072687901,397.469916860725));
#58002=CARTESIAN_POINT('',(354.103663159699,-19.4720072687901,397.029435834866));
#58003=CARTESIAN_POINT('',(354.103663159699,-19.4720072687901,397.029435834866));
#58004=CARTESIAN_POINT('Origin',(381.148528861449,-19.4720072687901,397.469916860725));
#58005=CARTESIAN_POINT('Origin',(375.115917770968,-19.47200726879,445.000000551893));
#58006=CARTESIAN_POINT('',(348.293514664609,-19.47200726879,406.557519926939));
#58007=CARTESIAN_POINT('',(348.293514664609,-19.47200726879,406.557519926939));
#58008=CARTESIAN_POINT('',(346.804949058683,-19.47200726879,407.640200290488));
#58009=CARTESIAN_POINT('Origin',(375.115917770968,-19.47200726879,445.000000551893));
#58010=CARTESIAN_POINT('',(346.804949058683,-19.47200726879,407.640200290488));
#58011=CARTESIAN_POINT('Origin',(330.010855217635,-19.47200726879,428.843435808162));
#58012=CARTESIAN_POINT('',(341.871411623583,-19.47200726879,404.534055188714));
#58013=CARTESIAN_POINT('Origin',(330.010855217635,-19.47200726879,428.843435808162));
#58014=CARTESIAN_POINT('',(341.871411623583,-19.47200726879,404.534055188714));
#58015=CARTESIAN_POINT('Origin',(373.638914192836,-19.4720072687901,397.11138277388));
#58016=CARTESIAN_POINT('',(346.858109252615,-19.4720072687901,400.907073898524));
#58017=CARTESIAN_POINT('',(346.858109252615,-19.4720072687901,400.907073898524));
#58018=CARTESIAN_POINT('Origin',(373.638914192836,-19.4720072687901,397.11138277388));
#58019=CARTESIAN_POINT('Origin',(375.115917770968,-19.47200726879,445.000000551893));
#58020=CARTESIAN_POINT('',(342.61001406469,-19.47200726879,411.226758936108));
#58021=CARTESIAN_POINT('',(342.61001406469,-19.47200726879,411.226758936108));
#58022=CARTESIAN_POINT('',(341.309143694988,-19.47200726879,412.528972672017));
#58023=CARTESIAN_POINT('Origin',(375.115917770968,-19.47200726879,445.000000551893));
#58024=CARTESIAN_POINT('',(341.309143694988,-19.47200726879,412.528972672017));
#58025=CARTESIAN_POINT('Origin',(328.038729822654,-19.47200726879,436.098336261576));
#58026=CARTESIAN_POINT('',(335.950438145117,-19.47200726879,410.232844660214));
#58027=CARTESIAN_POINT('Origin',(328.038729822654,-19.47200726879,436.098336261576));
#58028=CARTESIAN_POINT('',(335.950438145117,-19.47200726879,410.232844660214));
#58029=CARTESIAN_POINT('Origin',(366.16566825421,-19.4720072687901,397.93202538994));
#58030=CARTESIAN_POINT('',(340.308356373543,-19.47200726879,405.870426152421));
#58031=CARTESIAN_POINT('',(340.308356373543,-19.47200726879,405.870426152421));
#58032=CARTESIAN_POINT('Origin',(366.16566825421,-19.4720072687901,397.93202538994));
#58033=CARTESIAN_POINT('Origin',(375.115917770968,-19.47200726879,445.000000551893));
#58034=CARTESIAN_POINT('',(337.726916694929,-19.47200726879,416.72760724082));
#58035=CARTESIAN_POINT('',(337.726916694929,-19.47200726879,416.72760724082));
#58036=CARTESIAN_POINT('',(336.645773307294,-19.47200726879,418.217289525112));
#58037=CARTESIAN_POINT('Origin',(375.115917770968,-19.47200726879,445.000000551893));
#58038=CARTESIAN_POINT('',(336.645773307294,-19.47200726879,418.217289525112));
#58039=CARTESIAN_POINT('Origin',(327.225801035189,-19.47200726879,443.572425232748));
#58040=CARTESIAN_POINT('',(330.993848757813,-19.47200726879,416.787716895342));
#58041=CARTESIAN_POINT('Origin',(327.225801035189,-19.47200726879,443.572425232748));
#58042=CARTESIAN_POINT('',(330.993848757813,-19.47200726879,416.787716895342));
#58043=CARTESIAN_POINT('Origin',(358.912807162862,-19.4720072687901,399.911637764141));
#58044=CARTESIAN_POINT('',(334.615681175749,-19.47200726879,411.797278391646));
#58045=CARTESIAN_POINT('',(334.615681175749,-19.47200726879,411.797278391646));
#58046=CARTESIAN_POINT('Origin',(358.912807162862,-19.4720072687901,399.911637764141));
#58047=CARTESIAN_POINT('Origin',(375.115917770968,-19.47200726879,445.000000551893));
#58048=CARTESIAN_POINT('',(333.764460618641,-19.47200726879,422.924615699545));
#58049=CARTESIAN_POINT('',(333.764460618641,-19.47200726879,422.924615699545));
#58050=CARTESIAN_POINT('',(332.929665551385,-19.47200726879,424.565085610408));
#58051=CARTESIAN_POINT('Origin',(375.115917770968,-19.47200726879,445.000000551893));
#58052=CARTESIAN_POINT('',(332.929665551385,-19.47200726879,424.565085610408));
#58053=CARTESIAN_POINT('Origin',(327.592085859944,-19.47200726879,451.081665846128));
#58054=CARTESIAN_POINT('',(327.123691142365,-19.47200726879,424.037269185296));
#58055=CARTESIAN_POINT('Origin',(327.592085859944,-19.47200726879,451.081665846128));
#58056=CARTESIAN_POINT('',(327.123691142365,-19.47200726879,424.037269185296));
#58057=CARTESIAN_POINT('Origin',(352.058920429727,-19.4720072687901,403.001475269873));
#58058=CARTESIAN_POINT('',(329.920256215508,-19.47200726879,418.541691843973));
#58059=CARTESIAN_POINT('',(329.920256215508,-19.47200726879,418.541691843973));
#58060=CARTESIAN_POINT('Origin',(352.058920429727,-19.4720072687901,403.001475269873));
#58061=CARTESIAN_POINT('Origin',(375.115917770968,-19.47200726879,445.000000551893));
#58062=CARTESIAN_POINT('',(330.820214655061,-19.47200726879,429.665193397337));
#58063=CARTESIAN_POINT('',(330.820214655061,-19.47200726879,429.665193397337));
#58064=CARTESIAN_POINT('',(330.252323333266,-19.47200726879,431.416057121158));
#58065=CARTESIAN_POINT('Origin',(375.115917770968,-19.47200726879,445.000000551893));
#58066=CARTESIAN_POINT('',(330.252323333266,-19.47200726879,431.416057121158));
#58067=CARTESIAN_POINT('Origin',(329.128565148903,-19.47200726879,458.441155676074));
#58068=CARTESIAN_POINT('',(324.435261423582,-19.47200726879,431.802993492812));
#58069=CARTESIAN_POINT('Origin',(329.128565148903,-19.47200726879,458.441155676074));
#58070=CARTESIAN_POINT('',(324.435261423582,-19.47200726879,431.802993492812));
#58071=CARTESIAN_POINT('Origin',(345.77277349292,-19.47200726879,407.125455853163));
#58072=CARTESIAN_POINT('',(326.337698438563,-19.47200726879,425.937596666782));
#58073=CARTESIAN_POINT('',(326.337698438563,-19.47200726879,425.937596666782));
#58074=CARTESIAN_POINT('Origin',(345.77277349292,-19.47200726879,407.125455853163));
#58075=CARTESIAN_POINT('Origin',(375.115917770968,-19.47200726879,445.000000551893));
#58076=CARTESIAN_POINT('',(328.966675911205,-19.47200726879,436.783364940581));
#58077=CARTESIAN_POINT('',(328.966675911205,-19.47200726879,436.783364940581));
#58078=CARTESIAN_POINT('',(328.679671703937,-19.47200726879,438.601510401696));
#58079=CARTESIAN_POINT('Origin',(375.115917770968,-19.47200726879,445.000000551893));
#58080=CARTESIAN_POINT('',(328.679671703937,-19.47200726879,438.601510401696));
#58081=CARTESIAN_POINT('Origin',(331.797405682692,-19.47200726879,465.469679658226));
#58082=CARTESIAN_POINT('',(322.994757663527,-19.47200726879,439.893671912479));
#58083=CARTESIAN_POINT('Origin',(331.797405682692,-19.47200726879,465.469679658226));
#58084=CARTESIAN_POINT('',(322.994757663527,-19.47200726879,439.893671912479));
#58085=CARTESIAN_POINT('Origin',(340.209152152551,-19.47200726879,412.182033425343));
#58086=CARTESIAN_POINT('',(323.956222307212,-19.47200726879,433.802881137733));
#58087=CARTESIAN_POINT('',(323.956222307212,-19.47200726879,433.802881137733));
#58088=CARTESIAN_POINT('Origin',(340.209152152551,-19.47200726879,412.182033425343));
#58089=CARTESIAN_POINT('Origin',(375.115917770968,-19.47200726879,445.000000551893));
#58090=CARTESIAN_POINT('',(328.249484662489,-19.47200726879,444.103857322026));
#58091=CARTESIAN_POINT('',(328.249484662489,-19.47200726879,444.103857322026));
#58092=CARTESIAN_POINT('',(328.250434565844,-19.47200726879,445.944515745103));
#58093=CARTESIAN_POINT('Origin',(375.115917770968,-19.47200726879,445.000000551893));
#58094=CARTESIAN_POINT('',(328.250434565844,-19.47200726879,445.944515745103));
#58095=CARTESIAN_POINT('Origin',(335.532891749993,-19.47200726879,471.994172205811));
#58096=CARTESIAN_POINT('',(322.837649845529,-19.47200726879,448.11008509018));
#58097=CARTESIAN_POINT('Origin',(335.532891749993,-19.47200726879,471.994172205811));
#58098=CARTESIAN_POINT('',(322.837649845529,-19.47200726879,448.11008509018));
#58099=CARTESIAN_POINT('Origin',(335.50505123062,-19.47200726879,418.046698264767));
#58100=CARTESIAN_POINT('',(322.834467667472,-19.47200726879,441.943875849769));
#58101=CARTESIAN_POINT('',(322.834467667472,-19.47200726879,441.943875849769));
#58102=CARTESIAN_POINT('Origin',(335.50505123062,-19.47200726879,418.046698264767));
#58103=CARTESIAN_POINT('Origin',(375.115917770968,-19.47200726879,445.000000551893));
#58104=CARTESIAN_POINT('',(328.686300537678,-19.47200726879,451.446415723918));
#58105=CARTESIAN_POINT('',(328.686300537678,-19.47200726879,451.446415723918));
#58106=CARTESIAN_POINT('',(328.975181161882,-19.47200726879,453.264263989787));
#58107=CARTESIAN_POINT('Origin',(375.115917770968,-19.47200726879,445.000000551893));
#58108=CARTESIAN_POINT('',(328.975181161882,-19.47200726879,453.264263989787));
#58109=CARTESIAN_POINT('Origin',(340.243043286461,-19.47200726879,477.853978658756));
#58110=CARTESIAN_POINT('',(323.96780648548,-19.47200726879,456.24991766477));
#58111=CARTESIAN_POINT('Origin',(340.243043286461,-19.47200726879,477.853978658756));
#58112=CARTESIAN_POINT('',(323.96780648548,-19.47200726879,456.24991766477));
#58113=CARTESIAN_POINT('Origin',(331.776301303842,-19.47200726879,424.575042859381));
#58114=CARTESIAN_POINT('',(323.000055841466,-19.47200726879,450.160122494669));
#58115=CARTESIAN_POINT('',(323.000055841466,-19.47200726879,450.160122494669));
#58116=CARTESIAN_POINT('Origin',(331.776301303842,-19.47200726879,424.575042859381));
#58117=CARTESIAN_POINT('Origin',(375.115917770968,-19.47200726879,445.000000551893));
#58118=CARTESIAN_POINT('',(330.266367680215,-19.47200726879,458.630241989851));
#58119=CARTESIAN_POINT('',(330.266367680215,-19.47200726879,458.630241989851));
#58120=CARTESIAN_POINT('',(330.836065825561,-19.47200726879,460.380518641112));
#58121=CARTESIAN_POINT('Origin',(375.115917770968,-19.47200726879,445.000000551893));
#58122=CARTESIAN_POINT('',(330.836065825561,-19.47200726879,460.380518641112));
#58123=CARTESIAN_POINT('Origin',(345.811880729174,-19.47200726879,482.904811134609));
#58124=CARTESIAN_POINT('',(326.357399376129,-19.47200726879,464.112739943707));
#58125=CARTESIAN_POINT('Origin',(345.811880729174,-19.47200726879,482.904811134609));
#58126=CARTESIAN_POINT('',(326.357399376129,-19.47200726879,464.112739943707));
#58127=CARTESIAN_POINT('Origin',(329.114716570426,-19.47200726879,431.606317698934));
#58128=CARTESIAN_POINT('',(324.448909498793,-19.47200726879,458.249309811874));
#58129=CARTESIAN_POINT('',(324.448909498793,-19.47200726879,458.249309811874));
#58130=CARTESIAN_POINT('Origin',(329.114716570426,-19.47200726879,431.606317698934));
#58131=CARTESIAN_POINT('Origin',(375.115917770968,-19.47200726879,445.000000551893));
#58132=CARTESIAN_POINT('',(332.95077959311,-19.47200726879,465.478446475402));
#58133=CARTESIAN_POINT('',(332.95077959311,-19.47200726879,465.478446475402));
#58134=CARTESIAN_POINT('',(333.787267400539,-19.47200726879,467.118053892068));
#58135=CARTESIAN_POINT('Origin',(375.115917770968,-19.47200726879,445.000000551893));
#58136=CARTESIAN_POINT('',(333.787267400539,-19.47200726879,467.118053892068));
#58137=CARTESIAN_POINT('Origin',(352.102280818378,-19.47200726879,487.022301375061));
#58138=CARTESIAN_POINT('',(329.947588809904,-19.47200726879,471.504943147272));
#58139=CARTESIAN_POINT('Origin',(352.102280818378,-19.47200726879,487.022301375061));
#58140=CARTESIAN_POINT('',(329.947588809904,-19.47200726879,471.504943147272));
#58141=CARTESIAN_POINT('Origin',(327.5858340798,-19.47200726879,438.967389461411));
#58142=CARTESIAN_POINT('',(327.145353053941,-19.47200726879,466.012255163162));
#58143=CARTESIAN_POINT('',(327.145353053941,-19.47200726879,466.012255163162));
#58144=CARTESIAN_POINT('Origin',(327.5858340798,-19.47200726879,438.967389461411));
#58145=CARTESIAN_POINT('Origin',(375.115917770968,-19.47200726879,445.000000551893));
#58146=CARTESIAN_POINT('',(336.673437146014,-19.47200726879,471.822403658252));
#58147=CARTESIAN_POINT('',(336.673437146014,-19.47200726879,471.822403658252));
#58148=CARTESIAN_POINT('',(337.756117509564,-19.47200726879,473.310969264178));
#58149=CARTESIAN_POINT('Origin',(375.115917770968,-19.47200726879,445.000000551893));
#58150=CARTESIAN_POINT('',(337.756117509564,-19.47200726879,473.310969264178));
#58151=CARTESIAN_POINT('Origin',(358.959353027238,-19.47200726879,490.105063105225));
#58152=CARTESIAN_POINT('',(334.64997240779,-19.47200726879,478.244506699278));
#58153=CARTESIAN_POINT('Origin',(358.959353027238,-19.47200726879,490.105063105225));
#58154=CARTESIAN_POINT('',(334.64997240779,-19.47200726879,478.244506699278));
#58155=CARTESIAN_POINT('Origin',(327.227299992955,-19.47200726879,446.477004130025));
#58156=CARTESIAN_POINT('',(331.022991117599,-19.47200726879,473.257809070246));
#58157=CARTESIAN_POINT('',(331.022991117599,-19.47200726879,473.257809070246));
#58158=CARTESIAN_POINT('Origin',(327.227299992955,-19.47200726879,446.477004130025));
#58159=CARTESIAN_POINT('Origin',(375.115917770968,-19.47200726879,445.000000551893));
#58160=CARTESIAN_POINT('',(341.342676155183,-19.47200726879,477.505904258171));
#58161=CARTESIAN_POINT('',(341.342676155183,-19.47200726879,477.505904258171));
#58162=CARTESIAN_POINT('',(342.644889891093,-19.47200726879,478.806774627873));
#58163=CARTESIAN_POINT('Origin',(375.115917770968,-19.47200726879,445.000000551893));
#58164=CARTESIAN_POINT('',(342.644889891093,-19.47200726879,478.806774627873));
#58165=CARTESIAN_POINT('Origin',(366.214253480652,-19.47200726879,492.077188500207));
#58166=CARTESIAN_POINT('',(340.34876187929,-19.47200726879,484.165480177744));
#58167=CARTESIAN_POINT('Origin',(366.214253480652,-19.47200726879,492.077188500207));
#58168=CARTESIAN_POINT('',(340.34876187929,-19.47200726879,484.165480177744));
#58169=CARTESIAN_POINT('Origin',(328.047942609015,-19.47200726879,453.95025006865));
#58170=CARTESIAN_POINT('',(335.986343371497,-19.47200726879,479.807561949318));
#58171=CARTESIAN_POINT('',(335.986343371497,-19.47200726879,479.807561949318));
#58172=CARTESIAN_POINT('Origin',(328.047942609015,-19.47200726879,453.95025006865));
#58173=CARTESIAN_POINT('Origin',(375.115917770968,-19.47200726879,445.000000551893));
#58174=CARTESIAN_POINT('',(346.843524459896,-19.47200726879,482.389001627931));
#58175=CARTESIAN_POINT('',(346.843524459896,-19.47200726879,482.389001627931));
#58176=CARTESIAN_POINT('',(348.333206744188,-19.47200726879,483.470145015567));
#58177=CARTESIAN_POINT('Origin',(375.115917770968,-19.47200726879,445.000000551893));
#58178=CARTESIAN_POINT('',(348.333206744188,-19.47200726879,483.470145015567));
#58179=CARTESIAN_POINT('Origin',(373.688342451824,-19.47200726879,492.890117287672));
#58180=CARTESIAN_POINT('',(346.903634114418,-19.47200726879,489.122069565048));
#58181=CARTESIAN_POINT('Origin',(373.688342451824,-19.47200726879,492.890117287672));
#58182=CARTESIAN_POINT('',(346.903634114418,-19.47200726879,489.122069565048));
#58183=CARTESIAN_POINT('Origin',(330.027554983216,-19.47200726879,461.203111159998));
#58184=CARTESIAN_POINT('',(341.913195610722,-19.47200726879,485.500237147112));
#58185=CARTESIAN_POINT('',(341.913195610722,-19.47200726879,485.500237147112));
#58186=CARTESIAN_POINT('Origin',(330.027554983216,-19.47200726879,461.203111159998));
#58187=CARTESIAN_POINT('Origin',(375.115917770968,-19.47200726879,445.000000551893));
#58188=CARTESIAN_POINT('',(353.040532918621,-19.47200726879,486.35145770422));
#58189=CARTESIAN_POINT('',(353.040532918621,-19.47200726879,486.35145770422));
#58190=CARTESIAN_POINT('',(354.681002829484,-19.47200726879,487.186252771476));
#58191=CARTESIAN_POINT('Origin',(375.115917770968,-19.47200726879,445.000000551893));
#58192=CARTESIAN_POINT('',(354.681002829484,-19.47200726879,487.186252771476));
#58193=CARTESIAN_POINT('Origin',(381.197583065204,-19.47200726879,492.523832462917));
#58194=CARTESIAN_POINT('',(354.153186404372,-19.47200726879,492.992227180495));
#58195=CARTESIAN_POINT('Origin',(381.197583065204,-19.47200726879,492.523832462917));
#58196=CARTESIAN_POINT('',(354.153186404372,-19.47200726879,492.992227180495));
#58197=CARTESIAN_POINT('Origin',(333.117392488949,-19.47200726879,468.056997893134));
#58198=CARTESIAN_POINT('',(348.657609063049,-19.47200726879,490.195662107353));
#58199=CARTESIAN_POINT('',(348.657609063049,-19.47200726879,490.195662107353));
#58200=CARTESIAN_POINT('Origin',(333.117392488949,-19.47200726879,468.056997893134));
#58201=CARTESIAN_POINT('Origin',(375.115917770968,-19.47200726879,445.000000551893));
#58202=CARTESIAN_POINT('',(359.781110616413,-19.47200726879,489.2957036678));
#58203=CARTESIAN_POINT('',(359.781110616413,-19.47200726879,489.2957036678));
#58204=CARTESIAN_POINT('',(361.531974340233,-19.47200726879,489.863594989594));
#58205=CARTESIAN_POINT('Origin',(375.115917770968,-19.47200726879,445.000000551893));
#58206=CARTESIAN_POINT('',(361.531974340233,-19.47200726879,489.863594989594));
#58207=CARTESIAN_POINT('Origin',(388.55707289515,-19.47200726879,490.987353173957));
#58208=CARTESIAN_POINT('',(361.918910711888,-19.47200726879,495.680656899279));
#58209=CARTESIAN_POINT('Origin',(388.55707289515,-19.47200726879,490.987353173957));
#58210=CARTESIAN_POINT('',(361.918910711888,-19.47200726879,495.680656899279));
#58211=CARTESIAN_POINT('Origin',(337.241373072239,-19.47200726879,474.343144829941));
#58212=CARTESIAN_POINT('',(356.053513885857,-19.47200726879,493.778219884297));
#58213=CARTESIAN_POINT('',(356.053513885857,-19.47200726879,493.778219884297));
#58214=CARTESIAN_POINT('Origin',(337.241373072239,-19.47200726879,474.343144829941));
#58215=CARTESIAN_POINT('Origin',(375.115917770968,-19.47200726879,445.000000551893));
#58216=CARTESIAN_POINT('',(366.899282159657,-19.47200726879,491.149242411656));
#58217=CARTESIAN_POINT('',(366.899282159657,-19.47200726879,491.149242411656));
#58218=CARTESIAN_POINT('',(368.717427620771,-19.47200726879,491.436246618923));
#58219=CARTESIAN_POINT('Origin',(375.115917770968,-19.47200726879,445.000000551893));
#58220=CARTESIAN_POINT('',(368.717427620771,-19.47200726879,491.436246618923));
#58221=CARTESIAN_POINT('Origin',(395.585596877302,-19.47200726879,488.318512640169));
#58222=CARTESIAN_POINT('',(370.009589131554,-19.47200726879,497.121160659334));
#58223=CARTESIAN_POINT('Origin',(395.585596877302,-19.47200726879,488.318512640169));
#58224=CARTESIAN_POINT('',(370.009589131554,-19.47200726879,497.121160659334));
#58225=CARTESIAN_POINT('Origin',(342.297950644419,-19.47200726879,479.90676617031));
#58226=CARTESIAN_POINT('',(363.918798356808,-19.47200726879,496.159696015649));
#58227=CARTESIAN_POINT('',(363.918798356808,-19.47200726879,496.159696015649));
#58228=CARTESIAN_POINT('Origin',(342.297950644419,-19.47200726879,479.90676617031));
#58229=CARTESIAN_POINT('Origin',(375.115917770968,-19.47200726879,445.000000551893));
#58230=CARTESIAN_POINT('',(374.219774541101,-19.47200726879,491.866433660372));
#58231=CARTESIAN_POINT('',(374.219774541101,-19.47200726879,491.866433660372));
#58232=CARTESIAN_POINT('',(376.060432964178,-19.47200726879,491.865483757017));
#58233=CARTESIAN_POINT('Origin',(375.115917770968,-19.47200726879,445.000000551893));
#58234=CARTESIAN_POINT('',(376.060432964178,-19.47200726879,491.865483757017));
#58235=CARTESIAN_POINT('Origin',(402.110089424886,-19.47200726879,484.583026572868));
#58236=CARTESIAN_POINT('',(378.226002309256,-19.47200726879,497.278268477331));
#58237=CARTESIAN_POINT('Origin',(402.110089424886,-19.47200726879,484.583026572868));
#58238=CARTESIAN_POINT('',(378.226002309256,-19.47200726879,497.278268477331));
#58239=CARTESIAN_POINT('Origin',(348.162615483842,-19.47200726879,484.61086709224));
#58240=CARTESIAN_POINT('',(372.059793068845,-19.47200726879,497.281450655388));
#58241=CARTESIAN_POINT('',(372.059793068845,-19.47200726879,497.281450655388));
#58242=CARTESIAN_POINT('Origin',(348.162615483842,-19.47200726879,484.61086709224));
#58243=CARTESIAN_POINT('Origin',(375.115917770968,-19.47200726879,445.000000551893));
#58244=CARTESIAN_POINT('',(381.562332942994,-19.47200726879,491.429617785183));
#58245=CARTESIAN_POINT('',(381.562332942994,-19.47200726879,491.429617785183));
#58246=CARTESIAN_POINT('',(383.380181208862,-19.47200726879,491.140737160979));
#58247=CARTESIAN_POINT('Origin',(375.115917770968,-19.47200726879,445.000000551893));
#58248=CARTESIAN_POINT('',(383.380181208862,-19.47200726879,491.140737160979));
#58249=CARTESIAN_POINT('Origin',(407.969895877832,-19.47200726879,479.872875036399));
#58250=CARTESIAN_POINT('',(386.365834883846,-19.47200726879,496.14811183738));
#58251=CARTESIAN_POINT('Origin',(407.969895877832,-19.47200726879,479.872875036399));
#58252=CARTESIAN_POINT('',(386.365834883846,-19.47200726879,496.14811183738));
#58253=CARTESIAN_POINT('Origin',(354.690960078457,-19.47200726879,488.339617019018));
#58254=CARTESIAN_POINT('',(380.276039713744,-19.47200726879,497.115862481395));
#58255=CARTESIAN_POINT('',(380.276039713744,-19.47200726879,497.115862481395));
#58256=CARTESIAN_POINT('Origin',(354.690960078457,-19.47200726879,488.339617019018));
#58257=CARTESIAN_POINT('Origin',(375.115917770968,-19.47200726879,445.000000551893));
#58258=CARTESIAN_POINT('',(388.746159208926,-19.47200726879,489.849550642646));
#58259=CARTESIAN_POINT('',(388.746159208926,-19.47200726879,489.849550642646));
#58260=CARTESIAN_POINT('',(390.496435860187,-19.47200726879,489.2798524973));
#58261=CARTESIAN_POINT('Origin',(375.115917770968,-19.47200726879,445.000000551893));
#58262=CARTESIAN_POINT('',(390.496435860187,-19.47200726879,489.2798524973));
#58263=CARTESIAN_POINT('Origin',(413.020728353684,-19.47200726879,474.304037593687));
#58264=CARTESIAN_POINT('',(394.228657162783,-19.47200726879,493.758518946731));
#58265=CARTESIAN_POINT('Origin',(413.020728353684,-19.47200726879,474.304037593687));
#58266=CARTESIAN_POINT('',(394.228657162783,-19.47200726879,493.758518946731));
#58267=CARTESIAN_POINT('Origin',(361.72223491801,-19.47200726879,491.001201752435));
#58268=CARTESIAN_POINT('',(388.365227030949,-19.47200726879,495.667008824067));
#58269=CARTESIAN_POINT('',(388.365227030949,-19.47200726879,495.667008824067));
#58270=CARTESIAN_POINT('Origin',(361.72223491801,-19.47200726879,491.001201752435));
#58271=CARTESIAN_POINT('Origin',(375.115917770968,-19.47200726879,445.000000551893));
#58272=CARTESIAN_POINT('',(395.594363694478,-19.47200726879,487.165138729751));
#58273=CARTESIAN_POINT('',(395.594363694478,-19.47200726879,487.165138729751));
#58274=CARTESIAN_POINT('',(397.233971111143,-19.47200726879,486.328650922322));
#58275=CARTESIAN_POINT('Origin',(375.115917770968,-19.47200726879,445.000000551893));
#58276=CARTESIAN_POINT('',(397.233971111143,-19.47200726879,486.328650922322));
#58277=CARTESIAN_POINT('Origin',(417.138218594136,-19.47200726879,468.013637504482));
#58278=CARTESIAN_POINT('',(401.620860366348,-19.47200726879,490.168329512957));
#58279=CARTESIAN_POINT('Origin',(417.138218594136,-19.47200726879,468.013637504482));
#58280=CARTESIAN_POINT('',(401.620860366348,-19.47200726879,490.168329512957));
#58281=CARTESIAN_POINT('Origin',(369.083306680487,-19.47200726879,492.53008424306));
#58282=CARTESIAN_POINT('',(396.128172382238,-19.47200726879,492.970565268919));
#58283=CARTESIAN_POINT('',(396.128172382238,-19.47200726879,492.970565268919));
#58284=CARTESIAN_POINT('Origin',(369.083306680487,-19.47200726879,492.53008424306));
#58285=CARTESIAN_POINT('Origin',(375.115917770968,-19.47200726879,445.000000551893));
#58286=CARTESIAN_POINT('',(401.938320877327,-19.47200726879,483.442481176847));
#58287=CARTESIAN_POINT('',(401.938320877327,-19.47200726879,483.442481176847));
#58288=CARTESIAN_POINT('',(403.426886483253,-19.47200726879,482.359800813297));
#58289=CARTESIAN_POINT('Origin',(375.115917770968,-19.47200726879,445.000000551893));
#58290=CARTESIAN_POINT('',(403.426886483253,-19.47200726879,482.359800813297));
#58291=CARTESIAN_POINT('Origin',(420.220980324301,-19.47200726879,461.156565295623));
#58292=CARTESIAN_POINT('',(408.360423918353,-19.47200726879,485.465945915071));
#58293=CARTESIAN_POINT('Origin',(420.220980324301,-19.47200726879,461.156565295623));
#58294=CARTESIAN_POINT('',(408.360423918353,-19.47200726879,485.465945915071));
#58295=CARTESIAN_POINT('Origin',(376.5929213491,-19.47200726879,492.888618329905));
#58296=CARTESIAN_POINT('',(403.373726289321,-19.47200726879,489.092927205261));
#58297=CARTESIAN_POINT('',(403.373726289321,-19.47200726879,489.092927205261));
#58298=CARTESIAN_POINT('Origin',(376.5929213491,-19.47200726879,492.888618329905));
#58299=CARTESIAN_POINT('Origin',(375.115917770968,-19.47200726879,445.000000551893));
#58300=CARTESIAN_POINT('',(407.621821477246,-19.47200726879,478.773242167677));
#58301=CARTESIAN_POINT('',(407.621821477246,-19.47200726879,478.773242167677));
#58302=CARTESIAN_POINT('',(408.922691846948,-19.47200726879,477.471028431768));
#58303=CARTESIAN_POINT('Origin',(375.115917770968,-19.47200726879,445.000000551893));
#58304=CARTESIAN_POINT('',(408.922691846948,-19.47200726879,477.471028431768));
#58305=CARTESIAN_POINT('Origin',(422.193105719283,-19.47200726879,453.901664842209));
#58306=CARTESIAN_POINT('',(414.28139739682,-19.47200726879,479.767156443571));
#58307=CARTESIAN_POINT('Origin',(422.193105719283,-19.47200726879,453.901664842209));
#58308=CARTESIAN_POINT('',(414.28139739682,-19.47200726879,479.767156443571));
#58309=CARTESIAN_POINT('Origin',(384.066167287726,-19.47200726879,492.067975713845));
#58310=CARTESIAN_POINT('',(409.923479168393,-19.47200726879,484.129574951364));
#58311=CARTESIAN_POINT('',(409.923479168393,-19.47200726879,484.129574951364));
#58312=CARTESIAN_POINT('Origin',(384.066167287726,-19.47200726879,492.067975713845));
#58313=CARTESIAN_POINT('Origin',(375.115917770968,-19.47200726879,445.000000551893));
#58314=CARTESIAN_POINT('',(412.504918847007,-19.47200726879,473.272393862965));
#58315=CARTESIAN_POINT('',(412.504918847007,-19.47200726879,473.272393862965));
#58316=CARTESIAN_POINT('',(413.586062234642,-19.47200726879,471.782711578673));
#58317=CARTESIAN_POINT('Origin',(375.115917770968,-19.47200726879,445.000000551893));
#58318=CARTESIAN_POINT('',(413.586062234642,-19.47200726879,471.782711578673));
#58319=CARTESIAN_POINT('Origin',(423.006034506748,-19.4720072687901,446.427575871037));
#58320=CARTESIAN_POINT('',(419.237986784123,-19.47200726879,473.212284208443));
#58321=CARTESIAN_POINT('Origin',(423.006034506748,-19.4720072687901,446.427575871037));
#58322=CARTESIAN_POINT('',(419.237986784123,-19.47200726879,473.212284208443));
#58323=CARTESIAN_POINT('Origin',(391.319028379074,-19.47200726879,490.088363339644));
#58324=CARTESIAN_POINT('',(415.616154366188,-19.47200726879,478.202722712139));
#58325=CARTESIAN_POINT('',(415.616154366188,-19.47200726879,478.202722712139));
#58326=CARTESIAN_POINT('Origin',(391.319028379074,-19.47200726879,490.088363339644));
#58327=CARTESIAN_POINT('Origin',(375.115917770968,-19.47200726879,445.000000551893));
#58328=CARTESIAN_POINT('',(416.467374923295,-19.47200726879,467.07538540424));
#58329=CARTESIAN_POINT('',(416.467374923295,-19.47200726879,467.07538540424));
#58330=CARTESIAN_POINT('',(417.302169990551,-19.47200726879,465.434915493377));
#58331=CARTESIAN_POINT('Origin',(375.115917770968,-19.47200726879,445.000000551893));
#58332=CARTESIAN_POINT('',(417.302169990551,-19.47200726879,465.434915493377));
#58333=CARTESIAN_POINT('Origin',(422.639749681993,-19.4720072687901,438.918335257657));
#58334=CARTESIAN_POINT('',(423.108144399571,-19.47200726879,465.962731918489));
#58335=CARTESIAN_POINT('Origin',(422.639749681993,-19.4720072687901,438.918335257657));
#58336=CARTESIAN_POINT('',(423.108144399571,-19.47200726879,465.962731918489));
#58337=CARTESIAN_POINT('Origin',(398.17291511221,-19.47200726879,486.998525833912));
#58338=CARTESIAN_POINT('',(420.311579326428,-19.47200726879,471.458309259812));
#58339=CARTESIAN_POINT('',(420.311579326428,-19.47200726879,471.458309259812));
#58340=CARTESIAN_POINT('Origin',(398.17291511221,-19.47200726879,486.998525833912));
#58341=CARTESIAN_POINT('Origin',(375.115917770968,-19.47200726879,445.000000551893));
#58342=CARTESIAN_POINT('',(419.411620886875,-19.47200726879,460.334807706448));
#58343=CARTESIAN_POINT('',(419.411620886875,-19.47200726879,460.334807706448));
#58344=CARTESIAN_POINT('',(419.97951220867,-19.47200726879,458.583943982627));
#58345=CARTESIAN_POINT('Origin',(375.115917770968,-19.47200726879,445.000000551893));
#58346=CARTESIAN_POINT('',(419.97951220867,-19.47200726879,458.583943982627));
#58347=CARTESIAN_POINT('Origin',(421.103270393033,-19.4720072687901,431.558845427711));
#58348=CARTESIAN_POINT('',(425.796574118354,-19.47200726879,458.197007610973));
#58349=CARTESIAN_POINT('Origin',(421.103270393033,-19.4720072687901,431.558845427711));
#58350=CARTESIAN_POINT('',(425.796574118354,-19.47200726879,458.197007610973));
#58351=CARTESIAN_POINT('Origin',(404.459062049017,-19.47200726879,482.874545250622));
#58352=CARTESIAN_POINT('',(423.894137103373,-19.47200726879,464.062404437003));
#58353=CARTESIAN_POINT('',(423.894137103373,-19.47200726879,464.062404437003));
#58354=CARTESIAN_POINT('Origin',(404.459062049017,-19.47200726879,482.874545250622));
#58355=CARTESIAN_POINT('Origin',(375.115917770968,-19.47200726879,445.000000551893));
#58356=CARTESIAN_POINT('',(421.265159630731,-19.4720072687901,453.216636163204));
#58357=CARTESIAN_POINT('',(421.265159630731,-19.4720072687901,453.216636163204));
#58358=CARTESIAN_POINT('',(421.552163837999,-19.4720072687901,451.39849070209));
#58359=CARTESIAN_POINT('Origin',(375.115917770968,-19.47200726879,445.000000551893));
#58360=CARTESIAN_POINT('',(421.552163837999,-19.4720072687901,451.39849070209));
#58361=CARTESIAN_POINT('Origin',(418.434429859244,-19.4720072687901,424.530321445559));
#58362=CARTESIAN_POINT('',(427.23707787841,-19.4720072687901,450.106329191307));
#58363=CARTESIAN_POINT('Origin',(418.434429859244,-19.4720072687901,424.530321445559));
#58364=CARTESIAN_POINT('',(427.23707787841,-19.4720072687901,450.106329191307));
#58365=CARTESIAN_POINT('Origin',(410.022683389386,-19.47200726879,477.817967678442));
#58366=CARTESIAN_POINT('',(426.275613234725,-19.4720072687901,456.197119966052));
#58367=CARTESIAN_POINT('',(426.275613234725,-19.4720072687901,456.197119966052));
#58368=CARTESIAN_POINT('Origin',(410.022683389386,-19.47200726879,477.817967678442));
#58369=CARTESIAN_POINT('Origin',(375.115917770968,-19.47200726879,445.000000551893));
#58370=CARTESIAN_POINT('',(421.982350879447,-19.4720072687901,445.896143781759));
#58371=CARTESIAN_POINT('',(421.982350879447,-19.4720072687901,445.896143781759));
#58372=CARTESIAN_POINT('',(421.981400976092,-19.4720072687901,444.055485358683));
#58373=CARTESIAN_POINT('Origin',(375.115917770968,-19.47200726879,445.000000551893));
#58374=CARTESIAN_POINT('',(421.981400976092,-19.4720072687901,444.055485358683));
#58375=CARTESIAN_POINT('Origin',(414.698943791944,-19.4720072687901,418.005828897974));
#58376=CARTESIAN_POINT('',(427.394185696407,-19.4720072687901,441.889916013605));
#58377=CARTESIAN_POINT('Origin',(414.698943791944,-19.4720072687901,418.005828897974));
#58378=CARTESIAN_POINT('',(427.394185696407,-19.4720072687901,441.889916013605));
#58379=CARTESIAN_POINT('Origin',(414.726784311316,-19.47200726879,471.953302839018));
#58380=CARTESIAN_POINT('',(427.397367874464,-19.4720072687901,448.056125254016));
#58381=CARTESIAN_POINT('',(427.397367874464,-19.4720072687901,448.056125254016));
#58382=CARTESIAN_POINT('Origin',(414.726784311316,-19.47200726879,471.953302839018));
#58383=CARTESIAN_POINT('Origin',(375.115917770968,-19.47200726879,445.000000551893));
#58384=CARTESIAN_POINT('',(421.545535004259,-19.4720072687901,438.553585379867));
#58385=CARTESIAN_POINT('',(421.545535004259,-19.4720072687901,438.553585379867));
#58386=CARTESIAN_POINT('',(421.256654380055,-19.4720072687901,436.735737113998));
#58387=CARTESIAN_POINT('Origin',(375.115917770968,-19.47200726879,445.000000551893));
#58388=CARTESIAN_POINT('',(421.256654380055,-19.4720072687901,436.735737113998));
#58389=CARTESIAN_POINT('Origin',(409.988792255475,-19.4720072687901,412.146022445029));
#58390=CARTESIAN_POINT('',(426.264029056456,-19.4720072687901,433.750083439015));
#58391=CARTESIAN_POINT('Origin',(409.988792255475,-19.4720072687901,412.146022445029));
#58392=CARTESIAN_POINT('',(426.264029056456,-19.4720072687901,433.750083439015));
#58393=CARTESIAN_POINT('Origin',(418.455534238094,-19.47200726879,465.424958244404));
#58394=CARTESIAN_POINT('',(427.23177970047,-19.4720072687901,439.839878609116));
#58395=CARTESIAN_POINT('',(427.23177970047,-19.4720072687901,439.839878609116));
#58396=CARTESIAN_POINT('Origin',(418.455534238094,-19.47200726879,465.424958244404));
#58397=CARTESIAN_POINT('Origin',(375.115917770968,-19.47200726879,445.000000551893));
#58398=CARTESIAN_POINT('',(419.965467861721,-19.4720072687901,431.369759113934));
#58399=CARTESIAN_POINT('',(419.965467861721,-19.4720072687901,431.369759113934));
#58400=CARTESIAN_POINT('',(419.395769716375,-19.4720072687901,429.619482462673));
#58401=CARTESIAN_POINT('Origin',(375.115917770968,-19.47200726879,445.000000551893));
#58402=CARTESIAN_POINT('',(419.395769716375,-19.4720072687901,429.619482462673));
#58403=CARTESIAN_POINT('Origin',(404.419954812762,-19.4720072687901,407.095189969177));
#58404=CARTESIAN_POINT('',(423.874436165807,-19.4720072687901,425.887261160078));
#58405=CARTESIAN_POINT('Origin',(404.419954812762,-19.4720072687901,407.095189969177));
#58406=CARTESIAN_POINT('',(423.874436165807,-19.4720072687901,425.887261160078));
#58407=CARTESIAN_POINT('Origin',(421.117118971511,-19.47200726879,458.393683404851));
#58408=CARTESIAN_POINT('',(425.782926043143,-19.4720072687901,431.750691291911));
#58409=CARTESIAN_POINT('',(425.782926043143,-19.4720072687901,431.750691291911));
#58410=CARTESIAN_POINT('Origin',(421.117118971511,-19.47200726879,458.393683404851));
#58411=CARTESIAN_POINT('Origin',(375.115917770968,-19.47200726879,445.000000551893));
#58412=CARTESIAN_POINT('',(417.281055948826,-19.4720072687901,424.521554628383));
#58413=CARTESIAN_POINT('',(417.281055948826,-19.4720072687901,424.521554628383));
#58414=CARTESIAN_POINT('',(416.444568141397,-19.4720072687901,422.881947211718));
#58415=CARTESIAN_POINT('Origin',(375.115917770968,-19.47200726879,445.000000551893));
#58416=CARTESIAN_POINT('',(416.444568141397,-19.4720072687901,422.881947211718));
#58417=CARTESIAN_POINT('Origin',(398.129554723558,-19.4720072687901,402.977699728725));
#58418=CARTESIAN_POINT('',(420.284246732032,-19.4720072687901,418.495057956513));
#58419=CARTESIAN_POINT('Origin',(398.129554723558,-19.4720072687901,402.977699728725));
#58420=CARTESIAN_POINT('',(420.284246732032,-19.4720072687901,418.495057956513));
#58421=CARTESIAN_POINT('Origin',(422.646001462136,-19.4720072687901,451.032611642374));
#58422=CARTESIAN_POINT('',(423.086482487995,-19.4720072687901,423.987745940623));
#58423=CARTESIAN_POINT('',(423.086482487995,-19.4720072687901,423.987745940623));
#58424=CARTESIAN_POINT('Origin',(422.646001462136,-19.4720072687901,451.032611642374));
#58425=CARTESIAN_POINT('Origin',(375.115917770968,-19.47200726879,445.000000551893));
#58426=CARTESIAN_POINT('',(413.558398395922,-19.4720072687901,418.177597445533));
#58427=CARTESIAN_POINT('',(413.558398395922,-19.4720072687901,418.177597445533));
#58428=CARTESIAN_POINT('',(412.475718032372,-19.4720072687901,416.689031839608));
#58429=CARTESIAN_POINT('Origin',(375.115917770968,-19.47200726879,445.000000551893));
#58430=CARTESIAN_POINT('',(412.475718032372,-19.4720072687901,416.689031839608));
#58431=CARTESIAN_POINT('Origin',(391.272482514698,-19.4720072687901,399.89493799856));
#58432=CARTESIAN_POINT('',(415.581863134147,-19.4720072687901,411.755494404508));
#58433=CARTESIAN_POINT('Origin',(391.272482514698,-19.4720072687901,399.89493799856));
#58434=CARTESIAN_POINT('',(415.581863134147,-19.4720072687901,411.755494404508));
#58435=CARTESIAN_POINT('Origin',(423.004535548981,-19.4720072687901,443.522996973761));
#58436=CARTESIAN_POINT('',(419.208844424337,-19.4720072687901,416.742192033539));
#58437=CARTESIAN_POINT('',(419.208844424337,-19.4720072687901,416.742192033539));
#58438=CARTESIAN_POINT('Origin',(423.004535548981,-19.4720072687901,443.522996973761));
#58439=CARTESIAN_POINT('Origin',(375.115917770968,-19.47200726879,445.000000551893));
#58440=CARTESIAN_POINT('',(408.889159386753,-19.4720072687901,412.494096845614));
#58441=CARTESIAN_POINT('',(408.889159386753,-19.4720072687901,412.494096845614));
#58442=CARTESIAN_POINT('',(407.586945650843,-19.4720072687901,411.193226475912));
#58443=CARTESIAN_POINT('Origin',(375.115917770968,-19.47200726879,445.000000551893));
#58444=CARTESIAN_POINT('',(407.586945650843,-19.4720072687901,411.193226475912));
#58445=CARTESIAN_POINT('Origin',(384.017582061284,-19.4720072687901,397.922812603578));
#58446=CARTESIAN_POINT('',(409.883073662646,-19.4720072687901,405.834520926041));
#58447=CARTESIAN_POINT('Origin',(384.017582061284,-19.4720072687901,397.922812603578));
#58448=CARTESIAN_POINT('',(409.883073662646,-19.4720072687901,405.834520926041));
#58449=CARTESIAN_POINT('Origin',(422.183892932921,-19.4720072687901,436.049751035135));
#58450=CARTESIAN_POINT('',(414.245492170439,-19.4720072687901,410.192439154467));
#58451=CARTESIAN_POINT('',(414.245492170439,-19.4720072687901,410.192439154467));
#58452=CARTESIAN_POINT('Origin',(422.183892932921,-19.4720072687901,436.049751035135));
#58453=CARTESIAN_POINT('Origin',(375.115917770968,-19.47200726879,445.000000551893));
#58454=CARTESIAN_POINT('',(403.38831108204,-19.4720072687901,407.610999475854));
#58455=CARTESIAN_POINT('',(403.38831108204,-19.4720072687901,407.610999475854));
#58456=CARTESIAN_POINT('',(401.898628797749,-19.4720072687901,406.529856088218));
#58457=CARTESIAN_POINT('Origin',(375.115917770968,-19.47200726879,445.000000551893));
#58458=CARTESIAN_POINT('',(401.898628797749,-19.4720072687901,406.529856088218));
#58459=CARTESIAN_POINT('Origin',(376.543493090113,-19.4720072687901,397.109883816113));
#58460=CARTESIAN_POINT('',(403.328201427518,-19.4720072687901,400.877931538737));
#58461=CARTESIAN_POINT('Origin',(376.543493090113,-19.4720072687901,397.109883816113));
#58462=CARTESIAN_POINT('',(403.328201427518,-19.4720072687901,400.877931538737));
#58463=CARTESIAN_POINT('Origin',(420.20428055872,-19.4720072687901,428.796889943787));
#58464=CARTESIAN_POINT('',(408.318639931214,-19.4720072687901,404.499763956673));
#58465=CARTESIAN_POINT('',(408.318639931214,-19.4720072687901,404.499763956673));
#58466=CARTESIAN_POINT('Origin',(420.20428055872,-19.4720072687901,428.796889943787));
#58467=CARTESIAN_POINT('Origin',(375.115917770968,-19.47200726879,445.000000551893));
#58468=CARTESIAN_POINT('',(397.191302623315,-19.4720072687901,403.648543399565));
#58469=CARTESIAN_POINT('',(397.191302623315,-19.4720072687901,403.648543399565));
#58470=CARTESIAN_POINT('',(395.550832712453,-19.4720072687901,402.813748332309));
#58471=CARTESIAN_POINT('Origin',(375.115917770968,-19.47200726879,445.000000551893));
#58472=CARTESIAN_POINT('',(395.550832712453,-19.4720072687901,402.813748332309));
#58473=CARTESIAN_POINT('Origin',(369.034252476732,-19.4720072687901,397.476168640868));
#58474=CARTESIAN_POINT('',(396.078649137564,-19.4720072687901,397.00777392329));
#58475=CARTESIAN_POINT('Origin',(369.034252476732,-19.4720072687901,397.476168640868));
#58476=CARTESIAN_POINT('',(396.078649137564,-19.4720072687901,397.00777392329));
#58477=CARTESIAN_POINT('Origin',(417.114443052987,-19.4720072687901,421.943003210651));
#58478=CARTESIAN_POINT('',(401.574226478887,-19.4720072687901,399.804338996432));
#58479=CARTESIAN_POINT('',(401.574226478887,-19.4720072687901,399.804338996432));
#58480=CARTESIAN_POINT('Origin',(417.114443052987,-19.4720072687901,421.943003210651));
#58481=CARTESIAN_POINT('Origin',(375.115917770968,-19.47200726879,445.000000551893));
#58482=CARTESIAN_POINT('',(390.450724925524,-19.4720072687901,400.704297435985));
#58483=CARTESIAN_POINT('',(390.450724925524,-19.4720072687901,400.704297435985));
#58484=CARTESIAN_POINT('',(388.699861201703,-19.4720072687901,400.136406114191));
#58485=CARTESIAN_POINT('Origin',(375.115917770968,-19.47200726879,445.000000551893));
#58486=CARTESIAN_POINT('',(388.699861201703,-19.4720072687901,400.136406114191));
#58487=CARTESIAN_POINT('Origin',(361.674762646786,-19.4720072687901,399.012647929828));
#58488=CARTESIAN_POINT('',(388.312924830048,-19.4720072687901,394.319344204506));
#58489=CARTESIAN_POINT('Origin',(361.674762646786,-19.4720072687901,399.012647929828));
#58490=CARTESIAN_POINT('',(388.312924830048,-19.4720072687901,394.319344204506));
#58491=CARTESIAN_POINT('Origin',(412.990462469698,-19.4720072687901,415.656856273844));
#58492=CARTESIAN_POINT('',(394.178321656079,-19.4720072687901,396.221781219488));
#58493=CARTESIAN_POINT('',(394.178321656079,-19.4720072687901,396.221781219488));
#58494=CARTESIAN_POINT('Origin',(412.990462469698,-19.4720072687901,415.656856273844));
#58495=CARTESIAN_POINT('Origin',(375.115917770968,-19.47200726879,445.000000551893));
#58496=CARTESIAN_POINT('',(383.33255338228,-19.4720072687901,398.850758692129));
#58497=CARTESIAN_POINT('',(383.33255338228,-19.4720072687901,398.850758692129));
#58498=CARTESIAN_POINT('',(381.514407921165,-19.4720072687901,398.563754484862));
#58499=CARTESIAN_POINT('Origin',(375.115917770968,-19.47200726879,445.000000551893));
#58500=CARTESIAN_POINT('',(381.514407921165,-19.4720072687901,398.563754484862));
#58501=CARTESIAN_POINT('Origin',(354.646238664634,-19.4720072687901,401.681488463616));
#58502=CARTESIAN_POINT('',(380.222246410382,-19.4720072687901,392.878840444451));
#58503=CARTESIAN_POINT('Origin',(354.646238664634,-19.4720072687901,401.681488463616));
#58504=CARTESIAN_POINT('',(380.222246410382,-19.4720072687901,392.878840444451));
#58505=CARTESIAN_POINT('Origin',(407.933884897518,-19.4720072687901,410.093234933475));
#58506=CARTESIAN_POINT('',(386.313037185128,-19.4720072687901,393.840305088136));
#58507=CARTESIAN_POINT('',(386.313037185128,-19.4720072687901,393.840305088136));
#58508=CARTESIAN_POINT('Origin',(407.933884897518,-19.4720072687901,410.093234933475));
#58509=CARTESIAN_POINT('Origin',(375.115917770968,-19.47200726879,445.000000551893));
#58510=CARTESIAN_POINT('',(378.172042473091,-19.4720072687901,392.718550448397));
#58511=CARTESIAN_POINT('Origin',(375.115917770968,-19.47200726879,445.000000551893));
#58512=CARTESIAN_POINT('',(378.172042473091,-19.4720072687901,392.718550448397));
#58513=CARTESIAN_POINT('Origin',(375.115917770968,-19.47200726879,445.000000551893));
#58514=CARTESIAN_POINT('Origin',(375.115917770968,-19.47200726879,445.000000551893));
#58515=CARTESIAN_POINT('Origin',(375.115917770968,-19.47200726879,445.000000551893));
#58516=CARTESIAN_POINT('Origin',(375.115917770968,-19.47200726879,445.000000551893));
#58517=CARTESIAN_POINT('Origin',(375.115917770968,-19.47200726879,445.000000551893));
#58518=CARTESIAN_POINT('Origin',(375.115917770968,-19.47200726879,445.000000551893));
#58519=CARTESIAN_POINT('Origin',(375.115917770968,-19.47200726879,445.000000551893));
#58520=CARTESIAN_POINT('Origin',(375.115917770968,-19.47200726879,445.000000551893));
#58521=CARTESIAN_POINT('Origin',(375.115917770968,-19.47200726879,445.000000551893));
#58522=CARTESIAN_POINT('Origin',(375.115917770968,-19.47200726879,445.000000551893));
#58523=CARTESIAN_POINT('Origin',(375.115917770968,-19.47200726879,445.000000551893));
#58524=CARTESIAN_POINT('Origin',(375.115917770968,-19.47200726879,445.000000551893));
#58525=CARTESIAN_POINT('Origin',(375.115917770968,-19.47200726879,445.000000551893));
#58526=CARTESIAN_POINT('Origin',(375.115917770968,-19.47200726879,445.000000551893));
#58527=CARTESIAN_POINT('Origin',(375.115917770968,-19.47200726879,445.000000551893));
#58528=CARTESIAN_POINT('Origin',(375.115917770968,-19.47200726879,445.000000551893));
#58529=CARTESIAN_POINT('Origin',(375.115917770968,-19.47200726879,445.000000551893));
#58530=CARTESIAN_POINT('Origin',(375.115917770968,-19.47200726879,445.000000551893));
#58531=CARTESIAN_POINT('Origin',(375.115917770968,-19.47200726879,445.000000551893));
#58532=CARTESIAN_POINT('Origin',(375.115917770968,-19.47200726879,445.000000551893));
#58533=CARTESIAN_POINT('Origin',(375.115917770968,-19.47200726879,445.000000551893));
#58534=CARTESIAN_POINT('Origin',(375.115917770968,-19.47200726879,445.000000551893));
#58535=CARTESIAN_POINT('Origin',(375.115917770968,-19.47200726879,445.000000551893));
#58536=CARTESIAN_POINT('Origin',(375.115917770968,-19.47200726879,445.000000551893));
#58537=CARTESIAN_POINT('Origin',(375.115917770968,-19.47200726879,445.000000551893));
#58538=CARTESIAN_POINT('Origin',(375.115917770968,-19.47200726879,445.000000551893));
#58539=CARTESIAN_POINT('Origin',(375.115917770968,-19.47200726879,445.000000551893));
#58540=CARTESIAN_POINT('Origin',(375.115917770968,-19.47200726879,445.000000551893));
#58541=CARTESIAN_POINT('Origin',(375.115917770968,-19.47200726879,445.000000551893));
#58542=CARTESIAN_POINT('Origin',(375.115917770968,-19.47200726879,445.000000551893));
#58543=CARTESIAN_POINT('Origin',(375.115917770968,-19.47200726879,445.000000551893));
#58544=CARTESIAN_POINT('Origin',(375.115917770968,-19.47200726879,445.000000551893));
#58545=CARTESIAN_POINT('Origin',(375.115917770968,-19.47200726879,445.000000551893));
#58546=CARTESIAN_POINT('Origin',(375.115917770968,-19.47200726879,445.000000551893));
#58547=CARTESIAN_POINT('Origin',(375.115917770968,-19.47200726879,445.000000551893));
#58548=CARTESIAN_POINT('Origin',(375.115917770968,-19.47200726879,445.000000551893));
#58549=CARTESIAN_POINT('Origin',(375.115917770968,-19.47200726879,445.000000551893));
#58550=CARTESIAN_POINT('Origin',(375.115917770968,-19.47200726879,445.000000551893));
#58551=CARTESIAN_POINT('Origin',(375.115917770968,-19.47200726879,445.000000551893));
#58552=CARTESIAN_POINT('Origin',(375.115917770968,-19.47200726879,445.000000551893));
#58553=CARTESIAN_POINT('Origin',(375.115917770968,-19.47200726879,445.000000551893));
#58554=CARTESIAN_POINT('Origin',(375.115917770968,-19.47200726879,445.000000551893));
#58555=CARTESIAN_POINT('Origin',(375.115917770968,-19.47200726879,445.000000551893));
#58556=CARTESIAN_POINT('Origin',(375.115917770968,-19.47200726879,445.000000551893));
#58557=CARTESIAN_POINT('Origin',(375.115917770968,-19.47200726879,445.000000551893));
#58558=CARTESIAN_POINT('Origin',(375.115917770968,-19.47200726879,445.000000551893));
#58559=CARTESIAN_POINT('Origin',(375.115917770968,-19.47200726879,445.000000551893));
#58560=CARTESIAN_POINT('Origin',(375.115917770968,-19.47200726879,445.000000551893));
#58561=CARTESIAN_POINT('Origin',(375.115917770968,-19.47200726879,445.000000551893));
#58562=CARTESIAN_POINT('Origin',(375.115917770968,-19.47200726879,445.000000551893));
#58563=CARTESIAN_POINT('Origin',(375.115917770968,-19.47200726879,445.000000551893));
#58564=CARTESIAN_POINT('Origin',(375.115917770968,-19.47200726879,445.000000551893));
#58565=CARTESIAN_POINT('Origin',(375.115917770968,-19.47200726879,445.000000551893));
#58566=CARTESIAN_POINT('Origin',(375.115917770968,-19.47200726879,445.000000551893));
#58567=CARTESIAN_POINT('Origin',(375.115917770968,-19.47200726879,445.000000551893));
#58568=CARTESIAN_POINT('Origin',(375.115917770968,-19.47200726879,445.000000551893));
#58569=CARTESIAN_POINT('Origin',(375.115917770968,-19.47200726879,445.000000551893));
#58570=CARTESIAN_POINT('Origin',(375.115917770968,-19.47200726879,445.000000551893));
#58571=CARTESIAN_POINT('Origin',(375.115917770968,-19.47200726879,445.000000551893));
#58572=CARTESIAN_POINT('Origin',(375.115917770968,-19.47200726879,445.000000551893));
#58573=CARTESIAN_POINT('Origin',(375.115917770968,-19.47200726879,445.000000551893));
#58574=CARTESIAN_POINT('Origin',(375.115917770968,-19.47200726879,445.000000551893));
#58575=CARTESIAN_POINT('Origin',(375.115917770968,-19.47200726879,445.000000551893));
#58576=CARTESIAN_POINT('Origin',(375.115917770968,-19.47200726879,445.000000551893));
#58577=CARTESIAN_POINT('Origin',(375.115917770968,-19.47200726879,445.000000551893));
#58578=CARTESIAN_POINT('Origin',(375.115917770968,-19.47200726879,445.000000551893));
#58579=CARTESIAN_POINT('Origin',(375.115917770968,-19.47200726879,445.000000551893));
#58580=CARTESIAN_POINT('Origin',(375.115917770968,-19.47200726879,445.000000551893));
#58581=CARTESIAN_POINT('Origin',(375.115917770968,-19.47200726879,445.000000551893));
#58582=CARTESIAN_POINT('Origin',(375.115917770968,-19.47200726879,445.000000551893));
#58583=CARTESIAN_POINT('Origin',(375.115917770968,-19.47200726879,445.000000551893));
#58584=CARTESIAN_POINT('Origin',(375.115917770968,-19.47200726879,445.000000551893));
#58585=CARTESIAN_POINT('Origin',(375.115917770968,-19.47200726879,445.000000551893));
#58586=CARTESIAN_POINT('Origin',(375.115917770968,-19.47200726879,445.000000551893));
#58587=CARTESIAN_POINT('Origin',(375.115917770968,-19.47200726879,445.000000551893));
#58588=CARTESIAN_POINT('Origin',(375.115917770968,-19.47200726879,445.000000551893));
#58589=CARTESIAN_POINT('Origin',(375.115917770968,-19.47200726879,445.000000551893));
#58590=CARTESIAN_POINT('',(376.012061000835,-19.4720072687901,398.133567443413));
#58591=CARTESIAN_POINT('',(376.012061000835,-19.4720072687901,398.133567443413));
#58592=CARTESIAN_POINT('',(374.171402577758,-19.4720072687901,398.134517346768));
#58593=CARTESIAN_POINT('Origin',(375.115917770968,-19.47200726879,445.000000551893));
#58594=CARTESIAN_POINT('',(374.171402577758,-19.4720072687901,398.134517346768));
#58595=CARTESIAN_POINT('Origin',(348.12174611705,-19.4720072687901,405.416974530917));
#58596=CARTESIAN_POINT('',(372.005833232681,-19.4720072687901,392.721732626454));
#58597=CARTESIAN_POINT('Origin',(348.12174611705,-19.4720072687901,405.416974530917));
#58598=CARTESIAN_POINT('',(372.005833232681,-19.4720072687901,392.721732626454));
#58599=CARTESIAN_POINT('Origin',(402.069220058094,-19.4720072687901,405.389134011545));
#58600=CARTESIAN_POINT('Origin',(402.069220058094,-19.4720072687901,405.389134011545));
#58601=CARTESIAN_POINT('Origin',(375.115917770968,-19.47200726879,445.000000551893));
#58602=CARTESIAN_POINT('Origin',(375.115917770968,-19.47200726879,445.000000551893));
#58603=CARTESIAN_POINT('Origin',(375.115917770968,-19.47200726879,445.000000551893));
#61776=UNCERTAINTY_MEASURE_WITH_UNIT(LENGTH_MEASURE(0.01),#61812,
'DISTANCE_ACCURACY_VALUE',
'Maximum model space distance between geometric entities at asserted c
onnectivities');
#61780=UNCERTAINTY_MEASURE_WITH_UNIT(LENGTH_MEASURE(0.01),#61812,
'DISTANCE_ACCURACY_VALUE',
'Maximum model space distance between geometric entities at asserted c
onnectivities');
#61807=(
GEOMETRIC_REPRESENTATION_CONTEXT(3)
GLOBAL_UNCERTAINTY_ASSIGNED_CONTEXT((#61776))
GLOBAL_UNIT_ASSIGNED_CONTEXT((#61812,#61814,#61815))
REPRESENTATION_CONTEXT('','3D')
);
#61811=(
GEOMETRIC_REPRESENTATION_CONTEXT(3)
GLOBAL_UNCERTAINTY_ASSIGNED_CONTEXT((#61780))
GLOBAL_UNIT_ASSIGNED_CONTEXT((#61812,#61814,#61815))
REPRESENTATION_CONTEXT('','3D')
);
#61812=(
LENGTH_UNIT()
NAMED_UNIT(*)
SI_UNIT(.MILLI.,.METRE.)
);
#61814=(
NAMED_UNIT(*)
PLANE_ANGLE_UNIT()
SI_UNIT($,.RADIAN.)
);
#61815=(
NAMED_UNIT(*)
SI_UNIT($,.STERADIAN.)
SOLID_ANGLE_UNIT()
);
#61842=SHAPE_DEFINITION_REPRESENTATION(#61904,#61994);
#61904=PRODUCT_DEFINITION_SHAPE('',$,#62025);
#61994=SHAPE_REPRESENTATION('',(#36744),#61807);
#61998=PRODUCT_DEFINITION_CONTEXT('part definition',#62090,'design');
#62025=PRODUCT_DEFINITION('Small Spur Gear','Small Spur Gear',#62055,#61998);
#62055=PRODUCT_DEFINITION_FORMATION('',$,#62118);
#62090=APPLICATION_CONTEXT('Managed model based 3d engineering');
#62091=PRODUCT_CONTEXT('part definition',#62090,'mechanical');
#62118=PRODUCT('Small Spur Gear','Small Spur Gear',$,(#62091));
#62143=COLOUR_RGB('Sky Blue',0.24,0.69,0.87);
#62144=FILL_AREA_STYLE_COLOUR('',#62143);
#62145=FILL_AREA_STYLE('',(#62144));
#62146=SURFACE_STYLE_FILL_AREA(#62145);
#62147=SURFACE_SIDE_STYLE('',(#62146));
#62148=SURFACE_STYLE_USAGE(.BOTH.,#62147);
#62149=PRESENTATION_STYLE_ASSIGNMENT((#62148));
ENDSEC;
END-ISO-10303-21;
